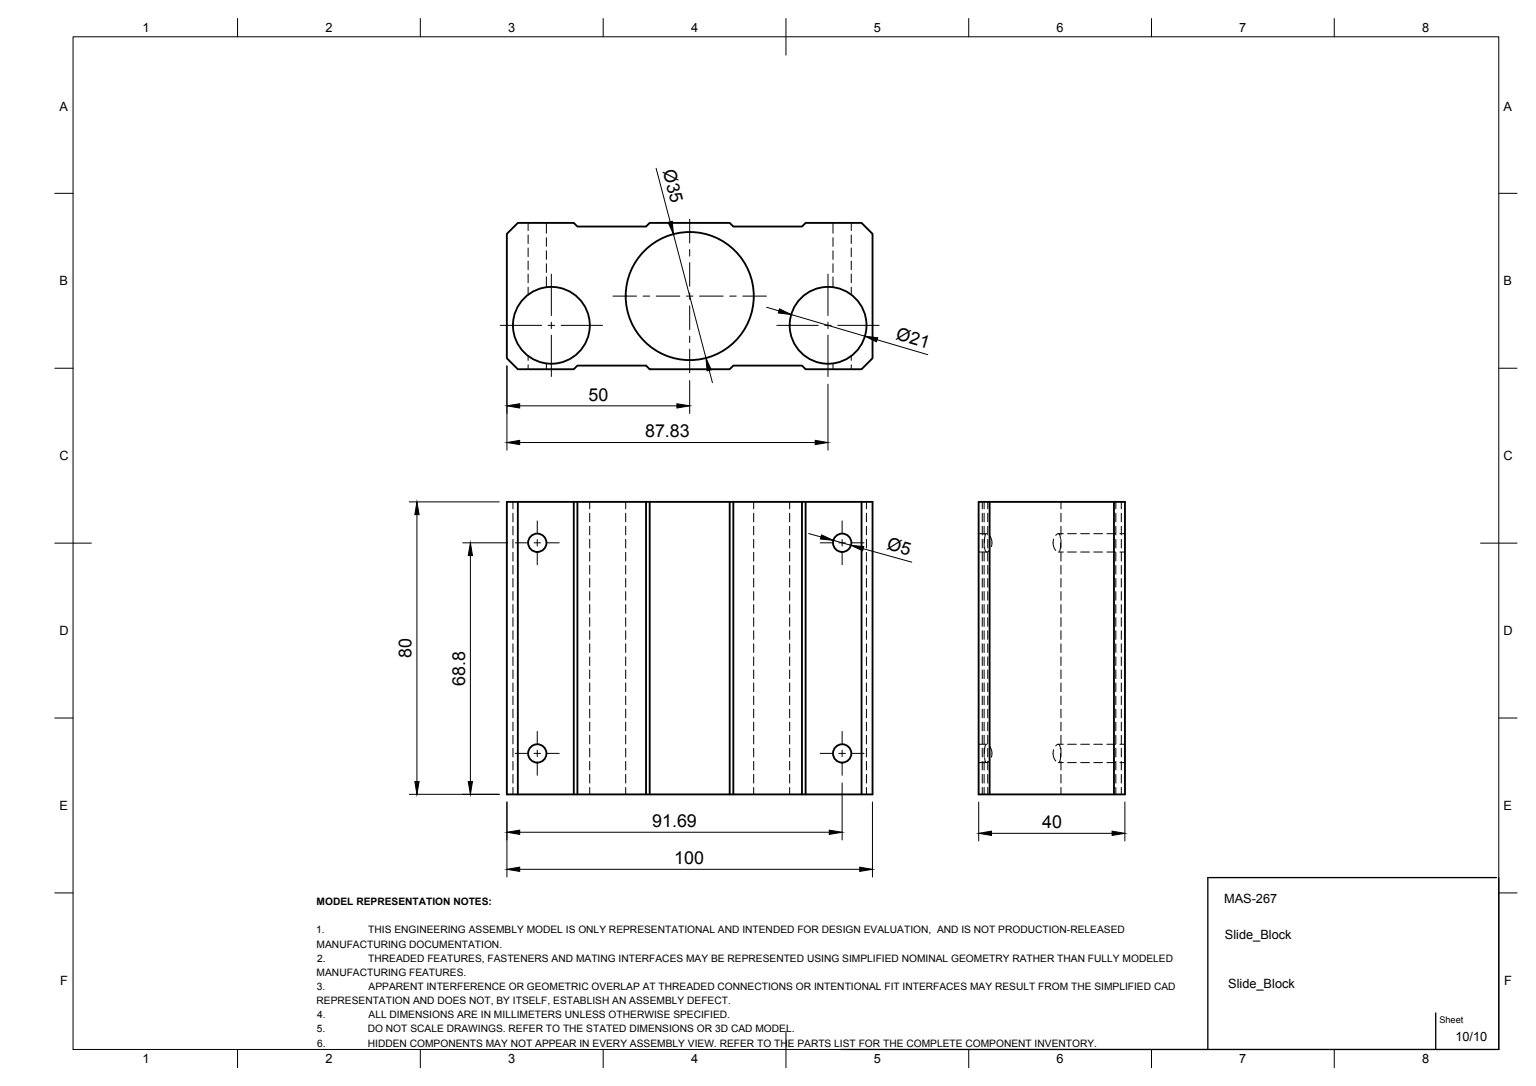
ISO-10303-21;
HEADER;
/* Generated by software containing ST-Developer
 * from STEP Tools, Inc. (www.steptools.com) 
 */

FILE_DESCRIPTION(
/* description */ (''),
/* implementation_level */ '2;1');

FILE_NAME(
/* name */ 'Slide_Block.step',
/* time_stamp */ '2026-10-12T15:29:24-07:00',
/* author */ (''),
/* organization */ (''),
/* preprocessor_version */ 'ST-DEVELOPER v20.2',
/* originating_system */ 'Autodesk Translation Framework v15.15.0.0',
/* authorisation */ '');

FILE_SCHEMA (('AUTOMOTIVE_DESIGN { 1 0 10303 214 3 1 1 }'));
ENDSEC;

DATA;
#10=MECHANICAL_DESIGN_GEOMETRIC_PRESENTATION_REPRESENTATION('',(#219),#9496);
#79=B_SPLINE_CURVE_WITH_KNOTS('',3,(#8964,#8965,#8966,#8967,#8968,#8969,
#8970,#8971,#8972,#8973),.UNSPECIFIED.,.F.,.F.,(4,2,2,2,4),(-1.57648415340294,
-1.48130138260372,-1.38611861180451,-1.27940954804234,-1.17270048428017),
 .UNSPECIFIED.);
#80=B_SPLINE_CURVE_WITH_KNOTS('',3,(#8974,#8975,#8976,#8977,#8978,#8979,
#8980,#8981,#8982,#8983,#8984,#8985,#8986,#8987,#8988,#8989,#8990,#8991,
#8992,#8993,#8994,#8995,#8996,#8997,#8998,#8999),.UNSPECIFIED.,.F.,.F.,
(4,2,2,2,2,2,2,2,2,2,2,2,4),(-1.17270048428017,-1.07435447096729,-0.976008457654416,
-0.882125267177943,-0.78824207670147,-0.694358886224997,-0.600475695748524,
-0.502129682435648,-0.403783669122773,-0.297074605360601,-0.190365541598429,
-0.0951827707992146,0.),.UNSPECIFIED.);
#81=B_SPLINE_CURVE_WITH_KNOTS('',3,(#9003,#9004,#9005,#9006,#9007,#9008,
#9009,#9010,#9011,#9012,#9013,#9014,#9015,#9016,#9017,#9018,#9019,#9020,
#9021,#9022,#9023,#9024,#9025,#9026,#9027,#9028),.UNSPECIFIED.,.F.,.F.,
(4,2,2,2,2,2,2,2,2,2,2,2,4),(-1.57648415340294,-1.48130138260372,-1.38611861180451,
-1.27940954804234,-1.17270048428017,-1.07435447096729,-0.976008457654416,
-0.882125267177943,-0.78824207670147,-0.694358886224997,-0.600475695748524,
-0.502129682435648,-0.403783669122773),.UNSPECIFIED.);
#82=B_SPLINE_CURVE_WITH_KNOTS('',3,(#9029,#9030,#9031,#9032,#9033,#9034,
#9035,#9036,#9037,#9038),.UNSPECIFIED.,.F.,.F.,(4,2,2,2,4),(-0.403783669122773,
-0.297074605360601,-0.190365541598429,-0.0951827707992147,0.),
 .UNSPECIFIED.);
#83=B_SPLINE_CURVE_WITH_KNOTS('',3,(#9048,#9049,#9050,#9051,#9052,#9053,
#9054,#9055,#9056,#9057,#9058,#9059,#9060,#9061,#9062,#9063,#9064,#9065,
#9066,#9067,#9068,#9069,#9070,#9071,#9072,#9073),.UNSPECIFIED.,.F.,.F.,
(4,2,2,2,2,2,2,2,2,2,2,2,4),(-1.57648415340294,-1.48130138260372,-1.38611861180451,
-1.27940954804234,-1.17270048428017,-1.07435447096729,-0.976008457654416,
-0.882125267177943,-0.78824207670147,-0.694358886224997,-0.600475695748524,
-0.502129682435648,-0.403783669122773),.UNSPECIFIED.);
#84=B_SPLINE_CURVE_WITH_KNOTS('',3,(#9074,#9075,#9076,#9077,#9078,#9079,
#9080,#9081,#9082,#9083),.UNSPECIFIED.,.F.,.F.,(4,2,2,2,4),(-0.403783669122773,
-0.297074605360601,-0.190365541598429,-0.0951827707992146,0.),
 .UNSPECIFIED.);
#85=B_SPLINE_CURVE_WITH_KNOTS('',3,(#9087,#9088,#9089,#9090,#9091,#9092,
#9093,#9094,#9095,#9096),.UNSPECIFIED.,.F.,.F.,(4,2,2,2,4),(-1.57648415340294,
-1.48130138260372,-1.38611861180451,-1.27940954804234,-1.17270048428017),
 .UNSPECIFIED.);
#86=B_SPLINE_CURVE_WITH_KNOTS('',3,(#9097,#9098,#9099,#9100,#9101,#9102,
#9103,#9104,#9105,#9106,#9107,#9108,#9109,#9110,#9111,#9112,#9113,#9114,
#9115,#9116,#9117,#9118,#9119,#9120,#9121,#9122),.UNSPECIFIED.,.F.,.F.,
(4,2,2,2,2,2,2,2,2,2,2,2,4),(-1.17270048428017,-1.07435447096729,-0.976008457654416,
-0.882125267177943,-0.78824207670147,-0.694358886224997,-0.600475695748524,
-0.502129682435648,-0.403783669122773,-0.297074605360601,-0.190365541598429,
-0.0951827707992147,0.),.UNSPECIFIED.);
#87=B_SPLINE_CURVE_WITH_KNOTS('',3,(#9132,#9133,#9134,#9135,#9136,#9137,
#9138,#9139,#9140,#9141),.UNSPECIFIED.,.F.,.F.,(4,2,2,2,4),(-1.57648415340294,
-1.48130138260372,-1.38611861180451,-1.27940954804234,-1.17270048428017),
 .UNSPECIFIED.);
#88=B_SPLINE_CURVE_WITH_KNOTS('',3,(#9142,#9143,#9144,#9145,#9146,#9147,
#9148,#9149,#9150,#9151,#9152,#9153,#9154,#9155,#9156,#9157,#9158,#9159,
#9160,#9161,#9162,#9163,#9164,#9165,#9166,#9167),.UNSPECIFIED.,.F.,.F.,
(4,2,2,2,2,2,2,2,2,2,2,2,4),(-1.17270048428017,-1.07435447096729,-0.976008457654416,
-0.882125267177943,-0.78824207670147,-0.694358886224997,-0.600475695748524,
-0.502129682435648,-0.403783669122773,-0.297074605360601,-0.190365541598429,
-0.0951827707992146,0.),.UNSPECIFIED.);
#89=B_SPLINE_CURVE_WITH_KNOTS('',3,(#9171,#9172,#9173,#9174,#9175,#9176,
#9177,#9178,#9179,#9180,#9181,#9182,#9183,#9184,#9185,#9186,#9187,#9188,
#9189,#9190,#9191,#9192,#9193,#9194,#9195,#9196),.UNSPECIFIED.,.F.,.F.,
(4,2,2,2,2,2,2,2,2,2,2,2,4),(-1.57648415340294,-1.48130138260372,-1.38611861180451,
-1.27940954804234,-1.17270048428017,-1.07435447096729,-0.976008457654416,
-0.882125267177943,-0.78824207670147,-0.694358886224997,-0.600475695748524,
-0.502129682435648,-0.403783669122773),.UNSPECIFIED.);
#90=B_SPLINE_CURVE_WITH_KNOTS('',3,(#9197,#9198,#9199,#9200,#9201,#9202,
#9203,#9204,#9205,#9206),.UNSPECIFIED.,.F.,.F.,(4,2,2,2,4),(-0.403783669122773,
-0.297074605360601,-0.190365541598429,-0.0951827707992147,0.),
 .UNSPECIFIED.);
#91=B_SPLINE_CURVE_WITH_KNOTS('',3,(#9216,#9217,#9218,#9219,#9220,#9221,
#9222,#9223,#9224,#9225,#9226,#9227,#9228,#9229,#9230,#9231,#9232,#9233,
#9234,#9235,#9236,#9237,#9238,#9239,#9240,#9241),.UNSPECIFIED.,.F.,.F.,
(4,2,2,2,2,2,2,2,2,2,2,2,4),(-1.57648415340294,-1.48130138260372,-1.38611861180451,
-1.27940954804234,-1.17270048428017,-1.07435447096729,-0.976008457654416,
-0.882125267177943,-0.78824207670147,-0.694358886224997,-0.600475695748524,
-0.502129682435648,-0.403783669122773),.UNSPECIFIED.);
#92=B_SPLINE_CURVE_WITH_KNOTS('',3,(#9242,#9243,#9244,#9245,#9246,#9247,
#9248,#9249,#9250,#9251),.UNSPECIFIED.,.F.,.F.,(4,2,2,2,4),(-0.403783669122773,
-0.297074605360601,-0.190365541598429,-0.0951827707992146,0.),
 .UNSPECIFIED.);
#93=B_SPLINE_CURVE_WITH_KNOTS('',3,(#9255,#9256,#9257,#9258,#9259,#9260,
#9261,#9262,#9263,#9264),.UNSPECIFIED.,.F.,.F.,(4,2,2,2,4),(-1.57648415340294,
-1.48130138260372,-1.38611861180451,-1.27940954804234,-1.17270048428017),
 .UNSPECIFIED.);
#94=B_SPLINE_CURVE_WITH_KNOTS('',3,(#9265,#9266,#9267,#9268,#9269,#9270,
#9271,#9272,#9273,#9274,#9275,#9276,#9277,#9278,#9279,#9280,#9281,#9282,
#9283,#9284,#9285,#9286,#9287,#9288,#9289,#9290),.UNSPECIFIED.,.F.,.F.,
(4,2,2,2,2,2,2,2,2,2,2,2,4),(-1.17270048428017,-1.07435447096729,-0.976008457654416,
-0.882125267177943,-0.78824207670147,-0.694358886224997,-0.600475695748524,
-0.502129682435648,-0.403783669122773,-0.297074605360601,-0.190365541598429,
-0.0951827707992147,0.),.UNSPECIFIED.);
#153=SHAPE_REPRESENTATION_RELATIONSHIP('SRR','None',#9547,#162);
#162=ADVANCED_BREP_SHAPE_REPRESENTATION('',(#276),#9495);
#219=STYLED_ITEM('',(#9593),#276);
#276=MANIFOLD_SOLID_BREP('Body1',#5021);
#460=FACE_BOUND('',#1388,.T.);
#461=FACE_BOUND('',#1389,.T.);
#462=FACE_BOUND('',#1392,.T.);
#463=FACE_BOUND('',#1393,.T.);
#464=FACE_BOUND('',#1394,.T.);
#465=FACE_BOUND('',#1399,.T.);
#466=FACE_BOUND('',#1400,.T.);
#467=FACE_BOUND('',#1401,.T.);
#468=FACE_BOUND('',#1403,.T.);
#469=FACE_BOUND('',#1404,.T.);
#470=FACE_BOUND('',#1409,.T.);
#471=FACE_BOUND('',#1410,.T.);
#472=FACE_BOUND('',#1416,.T.);
#473=FACE_BOUND('',#1417,.T.);
#474=FACE_BOUND('',#1419,.T.);
#475=FACE_BOUND('',#1420,.T.);
#476=FACE_BOUND('',#1421,.T.);
#477=FACE_BOUND('',#1422,.T.);
#478=FACE_BOUND('',#1424,.T.);
#479=FACE_BOUND('',#1425,.T.);
#480=FACE_BOUND('',#1426,.T.);
#481=FACE_BOUND('',#1427,.T.);
#596=PLANE('',#5774);
#597=PLANE('',#5775);
#598=PLANE('',#5776);
#599=PLANE('',#5777);
#600=PLANE('',#5778);
#601=PLANE('',#5779);
#602=PLANE('',#5783);
#603=PLANE('',#5784);
#604=PLANE('',#5785);
#605=PLANE('',#5786);
#606=PLANE('',#5790);
#607=PLANE('',#5791);
#608=PLANE('',#5792);
#609=PLANE('',#5793);
#610=PLANE('',#5794);
#611=PLANE('',#5795);
#612=PLANE('',#5796);
#613=PLANE('',#5797);
#614=PLANE('',#5798);
#615=PLANE('',#5799);
#616=PLANE('',#5803);
#617=PLANE('',#5804);
#618=PLANE('',#5805);
#619=PLANE('',#5806);
#620=PLANE('',#5807);
#621=PLANE('',#5808);
#917=FACE_OUTER_BOUND('',#1376,.T.);
#918=FACE_OUTER_BOUND('',#1377,.T.);
#919=FACE_OUTER_BOUND('',#1378,.T.);
#920=FACE_OUTER_BOUND('',#1379,.T.);
#921=FACE_OUTER_BOUND('',#1380,.T.);
#922=FACE_OUTER_BOUND('',#1381,.T.);
#923=FACE_OUTER_BOUND('',#1382,.T.);
#924=FACE_OUTER_BOUND('',#1383,.T.);
#925=FACE_OUTER_BOUND('',#1384,.T.);
#926=FACE_OUTER_BOUND('',#1385,.T.);
#927=FACE_OUTER_BOUND('',#1386,.T.);
#928=FACE_OUTER_BOUND('',#1387,.T.);
#929=FACE_OUTER_BOUND('',#1390,.T.);
#930=FACE_OUTER_BOUND('',#1391,.T.);
#931=FACE_OUTER_BOUND('',#1395,.T.);
#932=FACE_OUTER_BOUND('',#1396,.T.);
#933=FACE_OUTER_BOUND('',#1397,.T.);
#934=FACE_OUTER_BOUND('',#1398,.T.);
#935=FACE_OUTER_BOUND('',#1402,.T.);
#936=FACE_OUTER_BOUND('',#1405,.T.);
#937=FACE_OUTER_BOUND('',#1406,.T.);
#938=FACE_OUTER_BOUND('',#1407,.T.);
#939=FACE_OUTER_BOUND('',#1408,.T.);
#940=FACE_OUTER_BOUND('',#1411,.T.);
#941=FACE_OUTER_BOUND('',#1412,.T.);
#942=FACE_OUTER_BOUND('',#1413,.T.);
#943=FACE_OUTER_BOUND('',#1414,.T.);
#944=FACE_OUTER_BOUND('',#1415,.T.);
#945=FACE_OUTER_BOUND('',#1418,.T.);
#946=FACE_OUTER_BOUND('',#1423,.T.);
#947=FACE_OUTER_BOUND('',#1428,.T.);
#948=FACE_OUTER_BOUND('',#1429,.T.);
#949=FACE_OUTER_BOUND('',#1430,.T.);
#950=FACE_OUTER_BOUND('',#1431,.T.);
#951=FACE_OUTER_BOUND('',#1432,.T.);
#952=FACE_OUTER_BOUND('',#1433,.T.);
#953=FACE_OUTER_BOUND('',#1434,.T.);
#1376=EDGE_LOOP('',(#4319,#4320,#4321,#4322,#4323));
#1377=EDGE_LOOP('',(#4324,#4325,#4326,#4327,#4328));
#1378=EDGE_LOOP('',(#4329,#4330,#4331,#4332,#4333));
#1379=EDGE_LOOP('',(#4334,#4335,#4336,#4337,#4338));
#1380=EDGE_LOOP('',(#4339,#4340,#4341,#4342,#4343));
#1381=EDGE_LOOP('',(#4344,#4345,#4346,#4347,#4348));
#1382=EDGE_LOOP('',(#4349,#4350,#4351,#4352,#4353));
#1383=EDGE_LOOP('',(#4354,#4355,#4356,#4357,#4358));
#1384=EDGE_LOOP('',(#4359,#4360,#4361,#4362));
#1385=EDGE_LOOP('',(#4363,#4364,#4365,#4366));
#1386=EDGE_LOOP('',(#4367,#4368,#4369,#4370));
#1387=EDGE_LOOP('',(#4371,#4372,#4373,#4374));
#1388=EDGE_LOOP('',(#4375));
#1389=EDGE_LOOP('',(#4376));
#1390=EDGE_LOOP('',(#4377,#4378,#4379,#4380));
#1391=EDGE_LOOP('',(#4381,#4382,#4383,#4384,#4385,#4386,#4387,#4388,#4389,
#4390,#4391,#4392,#4393,#4394,#4395,#4396,#4397,#4398,#4399,#4400,#4401,
#4402,#4403,#4404));
#1392=EDGE_LOOP('',(#4405));
#1393=EDGE_LOOP('',(#4406));
#1394=EDGE_LOOP('',(#4407));
#1395=EDGE_LOOP('',(#4408,#4409,#4410,#4411));
#1396=EDGE_LOOP('',(#4412,#4413,#4414,#4415));
#1397=EDGE_LOOP('',(#4416,#4417,#4418,#4419));
#1398=EDGE_LOOP('',(#4420,#4421,#4422,#4423,#4424,#4425,#4426,#4427,#4428,
#4429,#4430,#4431,#4432,#4433,#4434,#4435,#4436,#4437,#4438,#4439,#4440,
#4441,#4442,#4443));
#1399=EDGE_LOOP('',(#4444));
#1400=EDGE_LOOP('',(#4445));
#1401=EDGE_LOOP('',(#4446));
#1402=EDGE_LOOP('',(#4447,#4448,#4449,#4450));
#1403=EDGE_LOOP('',(#4451));
#1404=EDGE_LOOP('',(#4452));
#1405=EDGE_LOOP('',(#4453,#4454,#4455,#4456));
#1406=EDGE_LOOP('',(#4457,#4458,#4459,#4460));
#1407=EDGE_LOOP('',(#4461,#4462,#4463,#4464));
#1408=EDGE_LOOP('',(#4465,#4466,#4467,#4468));
#1409=EDGE_LOOP('',(#4469));
#1410=EDGE_LOOP('',(#4470));
#1411=EDGE_LOOP('',(#4471,#4472,#4473,#4474));
#1412=EDGE_LOOP('',(#4475,#4476,#4477,#4478));
#1413=EDGE_LOOP('',(#4479,#4480,#4481,#4482));
#1414=EDGE_LOOP('',(#4483,#4484,#4485,#4486));
#1415=EDGE_LOOP('',(#4487,#4488,#4489,#4490));
#1416=EDGE_LOOP('',(#4491));
#1417=EDGE_LOOP('',(#4492));
#1418=EDGE_LOOP('',(#4493,#4494,#4495,#4496));
#1419=EDGE_LOOP('',(#4497,#4498));
#1420=EDGE_LOOP('',(#4499,#4500));
#1421=EDGE_LOOP('',(#4501,#4502));
#1422=EDGE_LOOP('',(#4503,#4504));
#1423=EDGE_LOOP('',(#4505,#4506,#4507,#4508));
#1424=EDGE_LOOP('',(#4509,#4510));
#1425=EDGE_LOOP('',(#4511,#4512));
#1426=EDGE_LOOP('',(#4513,#4514));
#1427=EDGE_LOOP('',(#4515,#4516));
#1428=EDGE_LOOP('',(#4517,#4518,#4519,#4520));
#1429=EDGE_LOOP('',(#4521,#4522,#4523,#4524));
#1430=EDGE_LOOP('',(#4525,#4526,#4527,#4528));
#1431=EDGE_LOOP('',(#4529,#4530,#4531,#4532));
#1432=EDGE_LOOP('',(#4533,#4534,#4535,#4536));
#1433=EDGE_LOOP('',(#4537,#4538,#4539,#4540));
#1434=EDGE_LOOP('',(#4541,#4542,#4543,#4544));
#1589=LINE('',#8962,#1826);
#1590=LINE('',#9040,#1827);
#1591=LINE('',#9046,#1828);
#1592=LINE('',#9124,#1829);
#1593=LINE('',#9130,#1830);
#1594=LINE('',#9208,#1831);
#1595=LINE('',#9214,#1832);
#1596=LINE('',#9292,#1833);
#1597=LINE('',#9297,#1834);
#1598=LINE('',#9299,#1835);
#1599=LINE('',#9301,#1836);
#1600=LINE('',#9302,#1837);
#1601=LINE('',#9305,#1838);
#1602=LINE('',#9307,#1839);
#1603=LINE('',#9308,#1840);
#1604=LINE('',#9311,#1841);
#1605=LINE('',#9313,#1842);
#1606=LINE('',#9314,#1843);
#1607=LINE('',#9317,#1844);
#1608=LINE('',#9319,#1845);
#1609=LINE('',#9320,#1846);
#1610=LINE('',#9323,#1847);
#1611=LINE('',#9325,#1848);
#1612=LINE('',#9326,#1849);
#1613=LINE('',#9329,#1850);
#1614=LINE('',#9331,#1851);
#1615=LINE('',#9333,#1852);
#1616=LINE('',#9335,#1853);
#1617=LINE('',#9337,#1854);
#1618=LINE('',#9339,#1855);
#1619=LINE('',#9341,#1856);
#1620=LINE('',#9343,#1857);
#1621=LINE('',#9345,#1858);
#1622=LINE('',#9347,#1859);
#1623=LINE('',#9349,#1860);
#1624=LINE('',#9351,#1861);
#1625=LINE('',#9353,#1862);
#1626=LINE('',#9355,#1863);
#1627=LINE('',#9357,#1864);
#1628=LINE('',#9359,#1865);
#1629=LINE('',#9361,#1866);
#1630=LINE('',#9363,#1867);
#1631=LINE('',#9364,#1868);
#1632=LINE('',#9373,#1869);
#1633=LINE('',#9375,#1870);
#1634=LINE('',#9376,#1871);
#1635=LINE('',#9379,#1872);
#1636=LINE('',#9380,#1873);
#1637=LINE('',#9382,#1874);
#1638=LINE('',#9385,#1875);
#1639=LINE('',#9387,#1876);
#1640=LINE('',#9389,#1877);
#1641=LINE('',#9391,#1878);
#1642=LINE('',#9393,#1879);
#1643=LINE('',#9395,#1880);
#1644=LINE('',#9397,#1881);
#1645=LINE('',#9399,#1882);
#1646=LINE('',#9401,#1883);
#1647=LINE('',#9403,#1884);
#1648=LINE('',#9405,#1885);
#1649=LINE('',#9407,#1886);
#1650=LINE('',#9409,#1887);
#1651=LINE('',#9411,#1888);
#1652=LINE('',#9413,#1889);
#1653=LINE('',#9414,#1890);
#1654=LINE('',#9422,#1891);
#1655=LINE('',#9424,#1892);
#1656=LINE('',#9425,#1893);
#1657=LINE('',#9427,#1894);
#1658=LINE('',#9429,#1895);
#1659=LINE('',#9431,#1896);
#1660=LINE('',#9433,#1897);
#1661=LINE('',#9435,#1898);
#1662=LINE('',#9436,#1899);
#1663=LINE('',#9438,#1900);
#1664=LINE('',#9441,#1901);
#1665=LINE('',#9443,#1902);
#1666=LINE('',#9445,#1903);
#1667=LINE('',#9447,#1904);
#1668=LINE('',#9449,#1905);
#1669=LINE('',#9451,#1906);
#1670=LINE('',#9454,#1907);
#1671=LINE('',#9456,#1908);
#1826=VECTOR('',#7256,2.5);
#1827=VECTOR('',#7259,2.5);
#1828=VECTOR('',#7266,2.5);
#1829=VECTOR('',#7269,2.5);
#1830=VECTOR('',#7276,2.5);
#1831=VECTOR('',#7279,2.5);
#1832=VECTOR('',#7286,2.5);
#1833=VECTOR('',#7289,2.5);
#1834=VECTOR('',#7294,10.);
#1835=VECTOR('',#7295,10.);
#1836=VECTOR('',#7296,10.);
#1837=VECTOR('',#7297,10.);
#1838=VECTOR('',#7300,10.);
#1839=VECTOR('',#7301,10.);
#1840=VECTOR('',#7302,10.);
#1841=VECTOR('',#7305,10.);
#1842=VECTOR('',#7306,10.);
#1843=VECTOR('',#7307,10.);
#1844=VECTOR('',#7310,10.);
#1845=VECTOR('',#7311,10.);
#1846=VECTOR('',#7312,10.);
#1847=VECTOR('',#7315,10.);
#1848=VECTOR('',#7316,10.);
#1849=VECTOR('',#7317,10.);
#1850=VECTOR('',#7320,10.);
#1851=VECTOR('',#7321,10.);
#1852=VECTOR('',#7322,10.);
#1853=VECTOR('',#7323,10.);
#1854=VECTOR('',#7324,10.);
#1855=VECTOR('',#7325,10.);
#1856=VECTOR('',#7326,10.);
#1857=VECTOR('',#7327,10.);
#1858=VECTOR('',#7328,10.);
#1859=VECTOR('',#7329,10.);
#1860=VECTOR('',#7330,10.);
#1861=VECTOR('',#7331,10.);
#1862=VECTOR('',#7332,10.);
#1863=VECTOR('',#7333,10.);
#1864=VECTOR('',#7334,10.);
#1865=VECTOR('',#7335,10.);
#1866=VECTOR('',#7336,10.);
#1867=VECTOR('',#7337,10.);
#1868=VECTOR('',#7338,10.);
#1869=VECTOR('',#7347,10.);
#1870=VECTOR('',#7348,10.);
#1871=VECTOR('',#7349,10.);
#1872=VECTOR('',#7352,10.);
#1873=VECTOR('',#7353,10.);
#1874=VECTOR('',#7356,10.);
#1875=VECTOR('',#7359,10.);
#1876=VECTOR('',#7360,10.);
#1877=VECTOR('',#7361,10.);
#1878=VECTOR('',#7362,10.);
#1879=VECTOR('',#7363,10.);
#1880=VECTOR('',#7364,10.);
#1881=VECTOR('',#7365,10.);
#1882=VECTOR('',#7366,10.);
#1883=VECTOR('',#7367,10.);
#1884=VECTOR('',#7368,10.);
#1885=VECTOR('',#7369,10.);
#1886=VECTOR('',#7370,10.);
#1887=VECTOR('',#7371,10.);
#1888=VECTOR('',#7372,10.);
#1889=VECTOR('',#7373,10.);
#1890=VECTOR('',#7374,10.);
#1891=VECTOR('',#7383,10.);
#1892=VECTOR('',#7386,10.);
#1893=VECTOR('',#7387,10.);
#1894=VECTOR('',#7390,10.);
#1895=VECTOR('',#7393,10.);
#1896=VECTOR('',#7396,10.);
#1897=VECTOR('',#7399,10.);
#1898=VECTOR('',#7402,10.);
#1899=VECTOR('',#7403,10.);
#1900=VECTOR('',#7406,10.);
#1901=VECTOR('',#7411,10.);
#1902=VECTOR('',#7414,10.5);
#1903=VECTOR('',#7417,10.5);
#1904=VECTOR('',#7420,17.5);
#1905=VECTOR('',#7423,10.);
#1906=VECTOR('',#7426,10.);
#1907=VECTOR('',#7431,10.);
#1908=VECTOR('',#7434,10.);
#2250=CIRCLE('',#5759,2.5);
#2251=CIRCLE('',#5761,2.5);
#2252=CIRCLE('',#5763,2.5);
#2253=CIRCLE('',#5765,2.5);
#2254=CIRCLE('',#5767,2.5);
#2255=CIRCLE('',#5769,2.5);
#2256=CIRCLE('',#5771,2.5);
#2257=CIRCLE('',#5773,2.5);
#2258=CIRCLE('',#5780,10.5);
#2259=CIRCLE('',#5781,10.5);
#2260=CIRCLE('',#5782,17.5);
#2261=CIRCLE('',#5787,10.5);
#2262=CIRCLE('',#5788,10.5);
#2263=CIRCLE('',#5789,17.5);
#2637=VERTEX_POINT('',#8959);
#2638=VERTEX_POINT('',#8961);
#2639=VERTEX_POINT('',#8963);
#2640=VERTEX_POINT('',#9001);
#2641=VERTEX_POINT('',#9002);
#2642=VERTEX_POINT('',#9039);
#2643=VERTEX_POINT('',#9043);
#2644=VERTEX_POINT('',#9045);
#2645=VERTEX_POINT('',#9047);
#2646=VERTEX_POINT('',#9085);
#2647=VERTEX_POINT('',#9086);
#2648=VERTEX_POINT('',#9123);
#2649=VERTEX_POINT('',#9127);
#2650=VERTEX_POINT('',#9129);
#2651=VERTEX_POINT('',#9131);
#2652=VERTEX_POINT('',#9169);
#2653=VERTEX_POINT('',#9170);
#2654=VERTEX_POINT('',#9207);
#2655=VERTEX_POINT('',#9211);
#2656=VERTEX_POINT('',#9213);
#2657=VERTEX_POINT('',#9215);
#2658=VERTEX_POINT('',#9253);
#2659=VERTEX_POINT('',#9254);
#2660=VERTEX_POINT('',#9291);
#2661=VERTEX_POINT('',#9295);
#2662=VERTEX_POINT('',#9296);
#2663=VERTEX_POINT('',#9298);
#2664=VERTEX_POINT('',#9300);
#2665=VERTEX_POINT('',#9304);
#2666=VERTEX_POINT('',#9306);
#2667=VERTEX_POINT('',#9310);
#2668=VERTEX_POINT('',#9312);
#2669=VERTEX_POINT('',#9316);
#2670=VERTEX_POINT('',#9318);
#2671=VERTEX_POINT('',#9322);
#2672=VERTEX_POINT('',#9324);
#2673=VERTEX_POINT('',#9328);
#2674=VERTEX_POINT('',#9330);
#2675=VERTEX_POINT('',#9332);
#2676=VERTEX_POINT('',#9334);
#2677=VERTEX_POINT('',#9336);
#2678=VERTEX_POINT('',#9338);
#2679=VERTEX_POINT('',#9340);
#2680=VERTEX_POINT('',#9342);
#2681=VERTEX_POINT('',#9344);
#2682=VERTEX_POINT('',#9346);
#2683=VERTEX_POINT('',#9348);
#2684=VERTEX_POINT('',#9350);
#2685=VERTEX_POINT('',#9352);
#2686=VERTEX_POINT('',#9354);
#2687=VERTEX_POINT('',#9356);
#2688=VERTEX_POINT('',#9358);
#2689=VERTEX_POINT('',#9360);
#2690=VERTEX_POINT('',#9362);
#2691=VERTEX_POINT('',#9365);
#2692=VERTEX_POINT('',#9367);
#2693=VERTEX_POINT('',#9369);
#2694=VERTEX_POINT('',#9372);
#2695=VERTEX_POINT('',#9374);
#2696=VERTEX_POINT('',#9378);
#2697=VERTEX_POINT('',#9384);
#2698=VERTEX_POINT('',#9386);
#2699=VERTEX_POINT('',#9388);
#2700=VERTEX_POINT('',#9390);
#2701=VERTEX_POINT('',#9392);
#2702=VERTEX_POINT('',#9394);
#2703=VERTEX_POINT('',#9396);
#2704=VERTEX_POINT('',#9398);
#2705=VERTEX_POINT('',#9400);
#2706=VERTEX_POINT('',#9402);
#2707=VERTEX_POINT('',#9404);
#2708=VERTEX_POINT('',#9406);
#2709=VERTEX_POINT('',#9408);
#2710=VERTEX_POINT('',#9410);
#2711=VERTEX_POINT('',#9412);
#2712=VERTEX_POINT('',#9415);
#2713=VERTEX_POINT('',#9417);
#2714=VERTEX_POINT('',#9419);
#3212=EDGE_CURVE('',#2637,#2637,#2250,.T.);
#3213=EDGE_CURVE('',#2637,#2638,#1589,.T.);
#3214=EDGE_CURVE('',#2639,#2638,#79,.T.);
#3215=EDGE_CURVE('',#2638,#2639,#80,.T.);
#3216=EDGE_CURVE('',#2640,#2641,#81,.T.);
#3217=EDGE_CURVE('',#2641,#2640,#82,.T.);
#3218=EDGE_CURVE('',#2641,#2642,#1590,.T.);
#3219=EDGE_CURVE('',#2642,#2642,#2251,.T.);
#3220=EDGE_CURVE('',#2643,#2643,#2252,.T.);
#3221=EDGE_CURVE('',#2643,#2644,#1591,.T.);
#3222=EDGE_CURVE('',#2645,#2644,#83,.T.);
#3223=EDGE_CURVE('',#2644,#2645,#84,.T.);
#3224=EDGE_CURVE('',#2646,#2647,#85,.T.);
#3225=EDGE_CURVE('',#2647,#2646,#86,.T.);
#3226=EDGE_CURVE('',#2647,#2648,#1592,.T.);
#3227=EDGE_CURVE('',#2648,#2648,#2253,.T.);
#3228=EDGE_CURVE('',#2649,#2649,#2254,.T.);
#3229=EDGE_CURVE('',#2649,#2650,#1593,.T.);
#3230=EDGE_CURVE('',#2651,#2650,#87,.T.);
#3231=EDGE_CURVE('',#2650,#2651,#88,.T.);
#3232=EDGE_CURVE('',#2652,#2653,#89,.T.);
#3233=EDGE_CURVE('',#2653,#2652,#90,.T.);
#3234=EDGE_CURVE('',#2653,#2654,#1594,.T.);
#3235=EDGE_CURVE('',#2654,#2654,#2255,.T.);
#3236=EDGE_CURVE('',#2655,#2655,#2256,.T.);
#3237=EDGE_CURVE('',#2655,#2656,#1595,.T.);
#3238=EDGE_CURVE('',#2657,#2656,#91,.T.);
#3239=EDGE_CURVE('',#2656,#2657,#92,.T.);
#3240=EDGE_CURVE('',#2658,#2659,#93,.T.);
#3241=EDGE_CURVE('',#2659,#2658,#94,.T.);
#3242=EDGE_CURVE('',#2659,#2660,#1596,.T.);
#3243=EDGE_CURVE('',#2660,#2660,#2257,.T.);
#3244=EDGE_CURVE('',#2661,#2662,#1597,.T.);
#3245=EDGE_CURVE('',#2661,#2663,#1598,.T.);
#3246=EDGE_CURVE('',#2664,#2663,#1599,.T.);
#3247=EDGE_CURVE('',#2662,#2664,#1600,.T.);
#3248=EDGE_CURVE('',#2665,#2661,#1601,.T.);
#3249=EDGE_CURVE('',#2665,#2666,#1602,.T.);
#3250=EDGE_CURVE('',#2663,#2666,#1603,.T.);
#3251=EDGE_CURVE('',#2667,#2665,#1604,.T.);
#3252=EDGE_CURVE('',#2668,#2667,#1605,.T.);
#3253=EDGE_CURVE('',#2666,#2668,#1606,.T.);
#3254=EDGE_CURVE('',#2664,#2669,#1607,.T.);
#3255=EDGE_CURVE('',#2670,#2669,#1608,.T.);
#3256=EDGE_CURVE('',#2670,#2662,#1609,.T.);
#3257=EDGE_CURVE('',#2667,#2671,#1610,.T.);
#3258=EDGE_CURVE('',#2671,#2672,#1611,.T.);
#3259=EDGE_CURVE('',#2672,#2668,#1612,.T.);
#3260=EDGE_CURVE('',#2673,#2670,#1613,.T.);
#3261=EDGE_CURVE('',#2673,#2674,#1614,.T.);
#3262=EDGE_CURVE('',#2675,#2674,#1615,.T.);
#3263=EDGE_CURVE('',#2676,#2675,#1616,.T.);
#3264=EDGE_CURVE('',#2676,#2677,#1617,.T.);
#3265=EDGE_CURVE('',#2677,#2678,#1618,.T.);
#3266=EDGE_CURVE('',#2678,#2679,#1619,.T.);
#3267=EDGE_CURVE('',#2680,#2679,#1620,.T.);
#3268=EDGE_CURVE('',#2680,#2681,#1621,.T.);
#3269=EDGE_CURVE('',#2681,#2682,#1622,.T.);
#3270=EDGE_CURVE('',#2682,#2683,#1623,.T.);
#3271=EDGE_CURVE('',#2684,#2683,#1624,.T.);
#3272=EDGE_CURVE('',#2685,#2684,#1625,.T.);
#3273=EDGE_CURVE('',#2686,#2685,#1626,.T.);
#3274=EDGE_CURVE('',#2687,#2686,#1627,.T.);
#3275=EDGE_CURVE('',#2688,#2687,#1628,.T.);
#3276=EDGE_CURVE('',#2688,#2689,#1629,.T.);
#3277=EDGE_CURVE('',#2689,#2690,#1630,.T.);
#3278=EDGE_CURVE('',#2690,#2671,#1631,.T.);
#3279=EDGE_CURVE('',#2691,#2691,#2258,.T.);
#3280=EDGE_CURVE('',#2692,#2692,#2259,.T.);
#3281=EDGE_CURVE('',#2693,#2693,#2260,.T.);
#3282=EDGE_CURVE('',#2694,#2688,#1632,.T.);
#3283=EDGE_CURVE('',#2695,#2694,#1633,.T.);
#3284=EDGE_CURVE('',#2689,#2695,#1634,.T.);
#3285=EDGE_CURVE('',#2696,#2695,#1635,.T.);
#3286=EDGE_CURVE('',#2690,#2696,#1636,.T.);
#3287=EDGE_CURVE('',#2672,#2696,#1637,.T.);
#3288=EDGE_CURVE('',#2697,#2694,#1638,.T.);
#3289=EDGE_CURVE('',#2698,#2697,#1639,.T.);
#3290=EDGE_CURVE('',#2699,#2698,#1640,.T.);
#3291=EDGE_CURVE('',#2700,#2699,#1641,.T.);
#3292=EDGE_CURVE('',#2701,#2700,#1642,.T.);
#3293=EDGE_CURVE('',#2701,#2702,#1643,.T.);
#3294=EDGE_CURVE('',#2702,#2703,#1644,.T.);
#3295=EDGE_CURVE('',#2703,#2704,#1645,.T.);
#3296=EDGE_CURVE('',#2705,#2704,#1646,.T.);
#3297=EDGE_CURVE('',#2705,#2706,#1647,.T.);
#3298=EDGE_CURVE('',#2706,#2707,#1648,.T.);
#3299=EDGE_CURVE('',#2707,#2708,#1649,.T.);
#3300=EDGE_CURVE('',#2709,#2708,#1650,.T.);
#3301=EDGE_CURVE('',#2710,#2709,#1651,.T.);
#3302=EDGE_CURVE('',#2711,#2710,#1652,.T.);
#3303=EDGE_CURVE('',#2669,#2711,#1653,.T.);
#3304=EDGE_CURVE('',#2712,#2712,#2261,.T.);
#3305=EDGE_CURVE('',#2713,#2713,#2262,.T.);
#3306=EDGE_CURVE('',#2714,#2714,#2263,.T.);
#3307=EDGE_CURVE('',#2697,#2687,#1654,.T.);
#3308=EDGE_CURVE('',#2708,#2676,#1655,.T.);
#3309=EDGE_CURVE('',#2677,#2707,#1656,.T.);
#3310=EDGE_CURVE('',#2678,#2706,#1657,.T.);
#3311=EDGE_CURVE('',#2679,#2705,#1658,.T.);
#3312=EDGE_CURVE('',#2709,#2675,#1659,.T.);
#3313=EDGE_CURVE('',#2704,#2680,#1660,.T.);
#3314=EDGE_CURVE('',#2682,#2702,#1661,.T.);
#3315=EDGE_CURVE('',#2683,#2701,#1662,.T.);
#3316=EDGE_CURVE('',#2681,#2703,#1663,.T.);
#3317=EDGE_CURVE('',#2684,#2700,#1664,.T.);
#3318=EDGE_CURVE('',#2691,#2712,#1665,.T.);
#3319=EDGE_CURVE('',#2713,#2692,#1666,.T.);
#3320=EDGE_CURVE('',#2714,#2693,#1667,.T.);
#3321=EDGE_CURVE('',#2686,#2698,#1668,.T.);
#3322=EDGE_CURVE('',#2699,#2685,#1669,.T.);
#3323=EDGE_CURVE('',#2711,#2673,#1670,.T.);
#3324=EDGE_CURVE('',#2674,#2710,#1671,.T.);
#4319=ORIENTED_EDGE('',*,*,#3212,.F.);
#4320=ORIENTED_EDGE('',*,*,#3213,.T.);
#4321=ORIENTED_EDGE('',*,*,#3214,.F.);
#4322=ORIENTED_EDGE('',*,*,#3215,.F.);
#4323=ORIENTED_EDGE('',*,*,#3213,.F.);
#4324=ORIENTED_EDGE('',*,*,#3216,.F.);
#4325=ORIENTED_EDGE('',*,*,#3217,.F.);
#4326=ORIENTED_EDGE('',*,*,#3218,.T.);
#4327=ORIENTED_EDGE('',*,*,#3219,.F.);
#4328=ORIENTED_EDGE('',*,*,#3218,.F.);
#4329=ORIENTED_EDGE('',*,*,#3220,.F.);
#4330=ORIENTED_EDGE('',*,*,#3221,.T.);
#4331=ORIENTED_EDGE('',*,*,#3222,.F.);
#4332=ORIENTED_EDGE('',*,*,#3223,.F.);
#4333=ORIENTED_EDGE('',*,*,#3221,.F.);
#4334=ORIENTED_EDGE('',*,*,#3224,.F.);
#4335=ORIENTED_EDGE('',*,*,#3225,.F.);
#4336=ORIENTED_EDGE('',*,*,#3226,.T.);
#4337=ORIENTED_EDGE('',*,*,#3227,.F.);
#4338=ORIENTED_EDGE('',*,*,#3226,.F.);
#4339=ORIENTED_EDGE('',*,*,#3228,.F.);
#4340=ORIENTED_EDGE('',*,*,#3229,.T.);
#4341=ORIENTED_EDGE('',*,*,#3230,.F.);
#4342=ORIENTED_EDGE('',*,*,#3231,.F.);
#4343=ORIENTED_EDGE('',*,*,#3229,.F.);
#4344=ORIENTED_EDGE('',*,*,#3232,.F.);
#4345=ORIENTED_EDGE('',*,*,#3233,.F.);
#4346=ORIENTED_EDGE('',*,*,#3234,.T.);
#4347=ORIENTED_EDGE('',*,*,#3235,.F.);
#4348=ORIENTED_EDGE('',*,*,#3234,.F.);
#4349=ORIENTED_EDGE('',*,*,#3236,.F.);
#4350=ORIENTED_EDGE('',*,*,#3237,.T.);
#4351=ORIENTED_EDGE('',*,*,#3238,.F.);
#4352=ORIENTED_EDGE('',*,*,#3239,.F.);
#4353=ORIENTED_EDGE('',*,*,#3237,.F.);
#4354=ORIENTED_EDGE('',*,*,#3240,.F.);
#4355=ORIENTED_EDGE('',*,*,#3241,.F.);
#4356=ORIENTED_EDGE('',*,*,#3242,.T.);
#4357=ORIENTED_EDGE('',*,*,#3243,.F.);
#4358=ORIENTED_EDGE('',*,*,#3242,.F.);
#4359=ORIENTED_EDGE('',*,*,#3244,.F.);
#4360=ORIENTED_EDGE('',*,*,#3245,.T.);
#4361=ORIENTED_EDGE('',*,*,#3246,.F.);
#4362=ORIENTED_EDGE('',*,*,#3247,.F.);
#4363=ORIENTED_EDGE('',*,*,#3248,.F.);
#4364=ORIENTED_EDGE('',*,*,#3249,.T.);
#4365=ORIENTED_EDGE('',*,*,#3250,.F.);
#4366=ORIENTED_EDGE('',*,*,#3245,.F.);
#4367=ORIENTED_EDGE('',*,*,#3251,.F.);
#4368=ORIENTED_EDGE('',*,*,#3252,.F.);
#4369=ORIENTED_EDGE('',*,*,#3253,.F.);
#4370=ORIENTED_EDGE('',*,*,#3249,.F.);
#4371=ORIENTED_EDGE('',*,*,#3247,.T.);
#4372=ORIENTED_EDGE('',*,*,#3254,.T.);
#4373=ORIENTED_EDGE('',*,*,#3255,.F.);
#4374=ORIENTED_EDGE('',*,*,#3256,.T.);
#4375=ORIENTED_EDGE('',*,*,#3219,.T.);
#4376=ORIENTED_EDGE('',*,*,#3235,.T.);
#4377=ORIENTED_EDGE('',*,*,#3252,.T.);
#4378=ORIENTED_EDGE('',*,*,#3257,.T.);
#4379=ORIENTED_EDGE('',*,*,#3258,.T.);
#4380=ORIENTED_EDGE('',*,*,#3259,.T.);
#4381=ORIENTED_EDGE('',*,*,#3251,.T.);
#4382=ORIENTED_EDGE('',*,*,#3248,.T.);
#4383=ORIENTED_EDGE('',*,*,#3244,.T.);
#4384=ORIENTED_EDGE('',*,*,#3256,.F.);
#4385=ORIENTED_EDGE('',*,*,#3260,.F.);
#4386=ORIENTED_EDGE('',*,*,#3261,.T.);
#4387=ORIENTED_EDGE('',*,*,#3262,.F.);
#4388=ORIENTED_EDGE('',*,*,#3263,.F.);
#4389=ORIENTED_EDGE('',*,*,#3264,.T.);
#4390=ORIENTED_EDGE('',*,*,#3265,.T.);
#4391=ORIENTED_EDGE('',*,*,#3266,.T.);
#4392=ORIENTED_EDGE('',*,*,#3267,.F.);
#4393=ORIENTED_EDGE('',*,*,#3268,.T.);
#4394=ORIENTED_EDGE('',*,*,#3269,.T.);
#4395=ORIENTED_EDGE('',*,*,#3270,.T.);
#4396=ORIENTED_EDGE('',*,*,#3271,.F.);
#4397=ORIENTED_EDGE('',*,*,#3272,.F.);
#4398=ORIENTED_EDGE('',*,*,#3273,.F.);
#4399=ORIENTED_EDGE('',*,*,#3274,.F.);
#4400=ORIENTED_EDGE('',*,*,#3275,.F.);
#4401=ORIENTED_EDGE('',*,*,#3276,.T.);
#4402=ORIENTED_EDGE('',*,*,#3277,.T.);
#4403=ORIENTED_EDGE('',*,*,#3278,.T.);
#4404=ORIENTED_EDGE('',*,*,#3257,.F.);
#4405=ORIENTED_EDGE('',*,*,#3279,.T.);
#4406=ORIENTED_EDGE('',*,*,#3280,.T.);
#4407=ORIENTED_EDGE('',*,*,#3281,.T.);
#4408=ORIENTED_EDGE('',*,*,#3276,.F.);
#4409=ORIENTED_EDGE('',*,*,#3282,.F.);
#4410=ORIENTED_EDGE('',*,*,#3283,.F.);
#4411=ORIENTED_EDGE('',*,*,#3284,.F.);
#4412=ORIENTED_EDGE('',*,*,#3277,.F.);
#4413=ORIENTED_EDGE('',*,*,#3284,.T.);
#4414=ORIENTED_EDGE('',*,*,#3285,.F.);
#4415=ORIENTED_EDGE('',*,*,#3286,.F.);
#4416=ORIENTED_EDGE('',*,*,#3278,.F.);
#4417=ORIENTED_EDGE('',*,*,#3286,.T.);
#4418=ORIENTED_EDGE('',*,*,#3287,.F.);
#4419=ORIENTED_EDGE('',*,*,#3258,.F.);
#4420=ORIENTED_EDGE('',*,*,#3253,.T.);
#4421=ORIENTED_EDGE('',*,*,#3259,.F.);
#4422=ORIENTED_EDGE('',*,*,#3287,.T.);
#4423=ORIENTED_EDGE('',*,*,#3285,.T.);
#4424=ORIENTED_EDGE('',*,*,#3283,.T.);
#4425=ORIENTED_EDGE('',*,*,#3288,.F.);
#4426=ORIENTED_EDGE('',*,*,#3289,.F.);
#4427=ORIENTED_EDGE('',*,*,#3290,.F.);
#4428=ORIENTED_EDGE('',*,*,#3291,.F.);
#4429=ORIENTED_EDGE('',*,*,#3292,.F.);
#4430=ORIENTED_EDGE('',*,*,#3293,.T.);
#4431=ORIENTED_EDGE('',*,*,#3294,.T.);
#4432=ORIENTED_EDGE('',*,*,#3295,.T.);
#4433=ORIENTED_EDGE('',*,*,#3296,.F.);
#4434=ORIENTED_EDGE('',*,*,#3297,.T.);
#4435=ORIENTED_EDGE('',*,*,#3298,.T.);
#4436=ORIENTED_EDGE('',*,*,#3299,.T.);
#4437=ORIENTED_EDGE('',*,*,#3300,.F.);
#4438=ORIENTED_EDGE('',*,*,#3301,.F.);
#4439=ORIENTED_EDGE('',*,*,#3302,.F.);
#4440=ORIENTED_EDGE('',*,*,#3303,.F.);
#4441=ORIENTED_EDGE('',*,*,#3254,.F.);
#4442=ORIENTED_EDGE('',*,*,#3246,.T.);
#4443=ORIENTED_EDGE('',*,*,#3250,.T.);
#4444=ORIENTED_EDGE('',*,*,#3304,.T.);
#4445=ORIENTED_EDGE('',*,*,#3305,.T.);
#4446=ORIENTED_EDGE('',*,*,#3306,.T.);
#4447=ORIENTED_EDGE('',*,*,#3282,.T.);
#4448=ORIENTED_EDGE('',*,*,#3275,.T.);
#4449=ORIENTED_EDGE('',*,*,#3307,.F.);
#4450=ORIENTED_EDGE('',*,*,#3288,.T.);
#4451=ORIENTED_EDGE('',*,*,#3227,.T.);
#4452=ORIENTED_EDGE('',*,*,#3243,.T.);
#4453=ORIENTED_EDGE('',*,*,#3264,.F.);
#4454=ORIENTED_EDGE('',*,*,#3308,.F.);
#4455=ORIENTED_EDGE('',*,*,#3299,.F.);
#4456=ORIENTED_EDGE('',*,*,#3309,.F.);
#4457=ORIENTED_EDGE('',*,*,#3265,.F.);
#4458=ORIENTED_EDGE('',*,*,#3309,.T.);
#4459=ORIENTED_EDGE('',*,*,#3298,.F.);
#4460=ORIENTED_EDGE('',*,*,#3310,.F.);
#4461=ORIENTED_EDGE('',*,*,#3266,.F.);
#4462=ORIENTED_EDGE('',*,*,#3310,.T.);
#4463=ORIENTED_EDGE('',*,*,#3297,.F.);
#4464=ORIENTED_EDGE('',*,*,#3311,.F.);
#4465=ORIENTED_EDGE('',*,*,#3308,.T.);
#4466=ORIENTED_EDGE('',*,*,#3263,.T.);
#4467=ORIENTED_EDGE('',*,*,#3312,.F.);
#4468=ORIENTED_EDGE('',*,*,#3300,.T.);
#4469=ORIENTED_EDGE('',*,*,#3212,.T.);
#4470=ORIENTED_EDGE('',*,*,#3228,.T.);
#4471=ORIENTED_EDGE('',*,*,#3311,.T.);
#4472=ORIENTED_EDGE('',*,*,#3296,.T.);
#4473=ORIENTED_EDGE('',*,*,#3313,.T.);
#4474=ORIENTED_EDGE('',*,*,#3267,.T.);
#4475=ORIENTED_EDGE('',*,*,#3270,.F.);
#4476=ORIENTED_EDGE('',*,*,#3314,.T.);
#4477=ORIENTED_EDGE('',*,*,#3293,.F.);
#4478=ORIENTED_EDGE('',*,*,#3315,.F.);
#4479=ORIENTED_EDGE('',*,*,#3269,.F.);
#4480=ORIENTED_EDGE('',*,*,#3316,.T.);
#4481=ORIENTED_EDGE('',*,*,#3294,.F.);
#4482=ORIENTED_EDGE('',*,*,#3314,.F.);
#4483=ORIENTED_EDGE('',*,*,#3268,.F.);
#4484=ORIENTED_EDGE('',*,*,#3313,.F.);
#4485=ORIENTED_EDGE('',*,*,#3295,.F.);
#4486=ORIENTED_EDGE('',*,*,#3316,.F.);
#4487=ORIENTED_EDGE('',*,*,#3315,.T.);
#4488=ORIENTED_EDGE('',*,*,#3292,.T.);
#4489=ORIENTED_EDGE('',*,*,#3317,.F.);
#4490=ORIENTED_EDGE('',*,*,#3271,.T.);
#4491=ORIENTED_EDGE('',*,*,#3220,.T.);
#4492=ORIENTED_EDGE('',*,*,#3236,.T.);
#4493=ORIENTED_EDGE('',*,*,#3279,.F.);
#4494=ORIENTED_EDGE('',*,*,#3318,.T.);
#4495=ORIENTED_EDGE('',*,*,#3304,.F.);
#4496=ORIENTED_EDGE('',*,*,#3318,.F.);
#4497=ORIENTED_EDGE('',*,*,#3224,.T.);
#4498=ORIENTED_EDGE('',*,*,#3225,.T.);
#4499=ORIENTED_EDGE('',*,*,#3222,.T.);
#4500=ORIENTED_EDGE('',*,*,#3223,.T.);
#4501=ORIENTED_EDGE('',*,*,#3240,.T.);
#4502=ORIENTED_EDGE('',*,*,#3241,.T.);
#4503=ORIENTED_EDGE('',*,*,#3238,.T.);
#4504=ORIENTED_EDGE('',*,*,#3239,.T.);
#4505=ORIENTED_EDGE('',*,*,#3305,.F.);
#4506=ORIENTED_EDGE('',*,*,#3319,.T.);
#4507=ORIENTED_EDGE('',*,*,#3280,.F.);
#4508=ORIENTED_EDGE('',*,*,#3319,.F.);
#4509=ORIENTED_EDGE('',*,*,#3216,.T.);
#4510=ORIENTED_EDGE('',*,*,#3217,.T.);
#4511=ORIENTED_EDGE('',*,*,#3214,.T.);
#4512=ORIENTED_EDGE('',*,*,#3215,.T.);
#4513=ORIENTED_EDGE('',*,*,#3232,.T.);
#4514=ORIENTED_EDGE('',*,*,#3233,.T.);
#4515=ORIENTED_EDGE('',*,*,#3230,.T.);
#4516=ORIENTED_EDGE('',*,*,#3231,.T.);
#4517=ORIENTED_EDGE('',*,*,#3306,.F.);
#4518=ORIENTED_EDGE('',*,*,#3320,.T.);
#4519=ORIENTED_EDGE('',*,*,#3281,.F.);
#4520=ORIENTED_EDGE('',*,*,#3320,.F.);
#4521=ORIENTED_EDGE('',*,*,#3289,.T.);
#4522=ORIENTED_EDGE('',*,*,#3307,.T.);
#4523=ORIENTED_EDGE('',*,*,#3274,.T.);
#4524=ORIENTED_EDGE('',*,*,#3321,.T.);
#4525=ORIENTED_EDGE('',*,*,#3321,.F.);
#4526=ORIENTED_EDGE('',*,*,#3273,.T.);
#4527=ORIENTED_EDGE('',*,*,#3322,.F.);
#4528=ORIENTED_EDGE('',*,*,#3290,.T.);
#4529=ORIENTED_EDGE('',*,*,#3272,.T.);
#4530=ORIENTED_EDGE('',*,*,#3317,.T.);
#4531=ORIENTED_EDGE('',*,*,#3291,.T.);
#4532=ORIENTED_EDGE('',*,*,#3322,.T.);
#4533=ORIENTED_EDGE('',*,*,#3260,.T.);
#4534=ORIENTED_EDGE('',*,*,#3255,.T.);
#4535=ORIENTED_EDGE('',*,*,#3303,.T.);
#4536=ORIENTED_EDGE('',*,*,#3323,.T.);
#4537=ORIENTED_EDGE('',*,*,#3323,.F.);
#4538=ORIENTED_EDGE('',*,*,#3302,.T.);
#4539=ORIENTED_EDGE('',*,*,#3324,.F.);
#4540=ORIENTED_EDGE('',*,*,#3261,.F.);
#4541=ORIENTED_EDGE('',*,*,#3301,.T.);
#4542=ORIENTED_EDGE('',*,*,#3312,.T.);
#4543=ORIENTED_EDGE('',*,*,#3262,.T.);
#4544=ORIENTED_EDGE('',*,*,#3324,.T.);
#4622=CYLINDRICAL_SURFACE('',#5758,2.5);
#4623=CYLINDRICAL_SURFACE('',#5760,2.5);
#4624=CYLINDRICAL_SURFACE('',#5762,2.5);
#4625=CYLINDRICAL_SURFACE('',#5764,2.5);
#4626=CYLINDRICAL_SURFACE('',#5766,2.5);
#4627=CYLINDRICAL_SURFACE('',#5768,2.5);
#4628=CYLINDRICAL_SURFACE('',#5770,2.5);
#4629=CYLINDRICAL_SURFACE('',#5772,2.5);
#4630=CYLINDRICAL_SURFACE('',#5800,10.5);
#4631=CYLINDRICAL_SURFACE('',#5801,10.5);
#4632=CYLINDRICAL_SURFACE('',#5802,17.5);
#4928=ADVANCED_FACE('',(#917),#4622,.F.);
#4929=ADVANCED_FACE('',(#918),#4623,.F.);
#4930=ADVANCED_FACE('',(#919),#4624,.F.);
#4931=ADVANCED_FACE('',(#920),#4625,.F.);
#4932=ADVANCED_FACE('',(#921),#4626,.F.);
#4933=ADVANCED_FACE('',(#922),#4627,.F.);
#4934=ADVANCED_FACE('',(#923),#4628,.F.);
#4935=ADVANCED_FACE('',(#924),#4629,.F.);
#4936=ADVANCED_FACE('',(#925),#596,.F.);
#4937=ADVANCED_FACE('',(#926),#597,.F.);
#4938=ADVANCED_FACE('',(#927),#598,.F.);
#4939=ADVANCED_FACE('',(#928,#460,#461),#599,.T.);
#4940=ADVANCED_FACE('',(#929),#600,.T.);
#4941=ADVANCED_FACE('',(#930,#462,#463,#464),#601,.T.);
#4942=ADVANCED_FACE('',(#931),#602,.T.);
#4943=ADVANCED_FACE('',(#932),#603,.T.);
#4944=ADVANCED_FACE('',(#933),#604,.T.);
#4945=ADVANCED_FACE('',(#934,#465,#466,#467),#605,.T.);
#4946=ADVANCED_FACE('',(#935,#468,#469),#606,.T.);
#4947=ADVANCED_FACE('',(#936),#607,.T.);
#4948=ADVANCED_FACE('',(#937),#608,.T.);
#4949=ADVANCED_FACE('',(#938),#609,.T.);
#4950=ADVANCED_FACE('',(#939,#470,#471),#610,.T.);
#4951=ADVANCED_FACE('',(#940),#611,.T.);
#4952=ADVANCED_FACE('',(#941),#612,.F.);
#4953=ADVANCED_FACE('',(#942),#613,.F.);
#4954=ADVANCED_FACE('',(#943),#614,.F.);
#4955=ADVANCED_FACE('',(#944,#472,#473),#615,.T.);
#4956=ADVANCED_FACE('',(#945,#474,#475,#476,#477),#4630,.F.);
#4957=ADVANCED_FACE('',(#946,#478,#479,#480,#481),#4631,.F.);
#4958=ADVANCED_FACE('',(#947),#4632,.F.);
#4959=ADVANCED_FACE('',(#948),#616,.T.);
#4960=ADVANCED_FACE('',(#949),#617,.T.);
#4961=ADVANCED_FACE('',(#950),#618,.T.);
#4962=ADVANCED_FACE('',(#951),#619,.T.);
#4963=ADVANCED_FACE('',(#952),#620,.T.);
#4964=ADVANCED_FACE('',(#953),#621,.T.);
#5021=CLOSED_SHELL('',(#4928,#4929,#4930,#4931,#4932,#4933,#4934,#4935,
#4936,#4937,#4938,#4939,#4940,#4941,#4942,#4943,#4944,#4945,#4946,#4947,
#4948,#4949,#4950,#4951,#4952,#4953,#4954,#4955,#4956,#4957,#4958,#4959,
#4960,#4961,#4962,#4963,#4964));
#5757=AXIS2_PLACEMENT_3D('',#8957,#7250,#7251);
#5758=AXIS2_PLACEMENT_3D('',#8958,#7252,#7253);
#5759=AXIS2_PLACEMENT_3D('',#8960,#7254,#7255);
#5760=AXIS2_PLACEMENT_3D('',#9000,#7257,#7258);
#5761=AXIS2_PLACEMENT_3D('',#9041,#7260,#7261);
#5762=AXIS2_PLACEMENT_3D('',#9042,#7262,#7263);
#5763=AXIS2_PLACEMENT_3D('',#9044,#7264,#7265);
#5764=AXIS2_PLACEMENT_3D('',#9084,#7267,#7268);
#5765=AXIS2_PLACEMENT_3D('',#9125,#7270,#7271);
#5766=AXIS2_PLACEMENT_3D('',#9126,#7272,#7273);
#5767=AXIS2_PLACEMENT_3D('',#9128,#7274,#7275);
#5768=AXIS2_PLACEMENT_3D('',#9168,#7277,#7278);
#5769=AXIS2_PLACEMENT_3D('',#9209,#7280,#7281);
#5770=AXIS2_PLACEMENT_3D('',#9210,#7282,#7283);
#5771=AXIS2_PLACEMENT_3D('',#9212,#7284,#7285);
#5772=AXIS2_PLACEMENT_3D('',#9252,#7287,#7288);
#5773=AXIS2_PLACEMENT_3D('',#9293,#7290,#7291);
#5774=AXIS2_PLACEMENT_3D('',#9294,#7292,#7293);
#5775=AXIS2_PLACEMENT_3D('',#9303,#7298,#7299);
#5776=AXIS2_PLACEMENT_3D('',#9309,#7303,#7304);
#5777=AXIS2_PLACEMENT_3D('',#9315,#7308,#7309);
#5778=AXIS2_PLACEMENT_3D('',#9321,#7313,#7314);
#5779=AXIS2_PLACEMENT_3D('',#9327,#7318,#7319);
#5780=AXIS2_PLACEMENT_3D('',#9366,#7339,#7340);
#5781=AXIS2_PLACEMENT_3D('',#9368,#7341,#7342);
#5782=AXIS2_PLACEMENT_3D('',#9370,#7343,#7344);
#5783=AXIS2_PLACEMENT_3D('',#9371,#7345,#7346);
#5784=AXIS2_PLACEMENT_3D('',#9377,#7350,#7351);
#5785=AXIS2_PLACEMENT_3D('',#9381,#7354,#7355);
#5786=AXIS2_PLACEMENT_3D('',#9383,#7357,#7358);
#5787=AXIS2_PLACEMENT_3D('',#9416,#7375,#7376);
#5788=AXIS2_PLACEMENT_3D('',#9418,#7377,#7378);
#5789=AXIS2_PLACEMENT_3D('',#9420,#7379,#7380);
#5790=AXIS2_PLACEMENT_3D('',#9421,#7381,#7382);
#5791=AXIS2_PLACEMENT_3D('',#9423,#7384,#7385);
#5792=AXIS2_PLACEMENT_3D('',#9426,#7388,#7389);
#5793=AXIS2_PLACEMENT_3D('',#9428,#7391,#7392);
#5794=AXIS2_PLACEMENT_3D('',#9430,#7394,#7395);
#5795=AXIS2_PLACEMENT_3D('',#9432,#7397,#7398);
#5796=AXIS2_PLACEMENT_3D('',#9434,#7400,#7401);
#5797=AXIS2_PLACEMENT_3D('',#9437,#7404,#7405);
#5798=AXIS2_PLACEMENT_3D('',#9439,#7407,#7408);
#5799=AXIS2_PLACEMENT_3D('',#9440,#7409,#7410);
#5800=AXIS2_PLACEMENT_3D('',#9442,#7412,#7413);
#5801=AXIS2_PLACEMENT_3D('',#9444,#7415,#7416);
#5802=AXIS2_PLACEMENT_3D('',#9446,#7418,#7419);
#5803=AXIS2_PLACEMENT_3D('',#9448,#7421,#7422);
#5804=AXIS2_PLACEMENT_3D('',#9450,#7424,#7425);
#5805=AXIS2_PLACEMENT_3D('',#9452,#7427,#7428);
#5806=AXIS2_PLACEMENT_3D('',#9453,#7429,#7430);
#5807=AXIS2_PLACEMENT_3D('',#9455,#7432,#7433);
#5808=AXIS2_PLACEMENT_3D('',#9457,#7435,#7436);
#7250=DIRECTION('axis',(0.,0.,1.));
#7251=DIRECTION('refdir',(1.,0.,0.));
#7252=DIRECTION('center_axis',(0.,0.,-1.));
#7253=DIRECTION('ref_axis',(-1.,0.,0.));
#7254=DIRECTION('center_axis',(0.,0.,-1.));
#7255=DIRECTION('ref_axis',(-1.,0.,0.));
#7256=DIRECTION('',(0.,0.,-1.));
#7257=DIRECTION('center_axis',(0.,0.,-1.));
#7258=DIRECTION('ref_axis',(-1.,0.,0.));
#7259=DIRECTION('',(0.,0.,-1.));
#7260=DIRECTION('center_axis',(0.,0.,1.));
#7261=DIRECTION('ref_axis',(-1.,0.,0.));
#7262=DIRECTION('center_axis',(0.,0.,-1.));
#7263=DIRECTION('ref_axis',(-1.,0.,0.));
#7264=DIRECTION('center_axis',(0.,0.,-1.));
#7265=DIRECTION('ref_axis',(-1.,0.,0.));
#7266=DIRECTION('',(0.,0.,-1.));
#7267=DIRECTION('center_axis',(0.,0.,-1.));
#7268=DIRECTION('ref_axis',(-1.,0.,0.));
#7269=DIRECTION('',(0.,0.,-1.));
#7270=DIRECTION('center_axis',(0.,0.,1.));
#7271=DIRECTION('ref_axis',(-1.,0.,0.));
#7272=DIRECTION('center_axis',(0.,0.,-1.));
#7273=DIRECTION('ref_axis',(-1.,0.,0.));
#7274=DIRECTION('center_axis',(0.,0.,-1.));
#7275=DIRECTION('ref_axis',(-1.,0.,0.));
#7276=DIRECTION('',(0.,0.,-1.));
#7277=DIRECTION('center_axis',(0.,0.,-1.));
#7278=DIRECTION('ref_axis',(-1.,0.,0.));
#7279=DIRECTION('',(0.,0.,-1.));
#7280=DIRECTION('center_axis',(0.,0.,1.));
#7281=DIRECTION('ref_axis',(-1.,0.,0.));
#7282=DIRECTION('center_axis',(0.,0.,-1.));
#7283=DIRECTION('ref_axis',(-1.,0.,0.));
#7284=DIRECTION('center_axis',(0.,0.,-1.));
#7285=DIRECTION('ref_axis',(-1.,0.,0.));
#7286=DIRECTION('',(0.,0.,-1.));
#7287=DIRECTION('center_axis',(0.,0.,-1.));
#7288=DIRECTION('ref_axis',(-1.,0.,0.));
#7289=DIRECTION('',(0.,0.,-1.));
#7290=DIRECTION('center_axis',(0.,0.,1.));
#7291=DIRECTION('ref_axis',(-1.,0.,0.));
#7292=DIRECTION('center_axis',(0.,-0.707106781186547,0.707106781186548));
#7293=DIRECTION('ref_axis',(0.,-0.707106781186548,-0.707106781186547));
#7294=DIRECTION('',(0.,-0.707106781186548,-0.707106781186547));
#7295=DIRECTION('',(1.,0.,0.));
#7296=DIRECTION('',(0.,0.707106781186548,0.707106781186547));
#7297=DIRECTION('',(1.,0.,0.));
#7298=DIRECTION('center_axis',(0.,0.,1.));
#7299=DIRECTION('ref_axis',(0.,-1.,0.));
#7300=DIRECTION('',(0.,-1.,0.));
#7301=DIRECTION('',(1.,0.,0.));
#7302=DIRECTION('',(0.,1.,0.));
#7303=DIRECTION('center_axis',(0.,0.707106781186548,0.707106781186548));
#7304=DIRECTION('ref_axis',(0.,-0.707106781186548,0.707106781186548));
#7305=DIRECTION('',(0.,-0.707106781186547,0.707106781186547));
#7306=DIRECTION('',(-1.,0.,0.));
#7307=DIRECTION('',(0.,0.707106781186547,-0.707106781186547));
#7308=DIRECTION('center_axis',(0.,0.,-1.));
#7309=DIRECTION('ref_axis',(-1.,0.,0.));
#7310=DIRECTION('',(0.,-1.,0.));
#7311=DIRECTION('',(1.,0.,0.));
#7312=DIRECTION('',(0.,1.,0.));
#7313=DIRECTION('center_axis',(0.,0.,-1.));
#7314=DIRECTION('ref_axis',(-1.,0.,0.));
#7315=DIRECTION('',(0.,1.,0.));
#7316=DIRECTION('',(1.,0.,0.));
#7317=DIRECTION('',(0.,-1.,0.));
#7318=DIRECTION('center_axis',(-1.,0.,0.));
#7319=DIRECTION('ref_axis',(0.,-1.,0.));
#7320=DIRECTION('',(0.,0.707106781186547,-0.707106781186548));
#7321=DIRECTION('',(0.,0.,1.));
#7322=DIRECTION('',(0.,-0.707106781186547,-0.707106781186548));
#7323=DIRECTION('',(0.,-1.,0.));
#7324=DIRECTION('',(0.,0.707106781186548,-0.707106781186547));
#7325=DIRECTION('',(0.,1.,0.));
#7326=DIRECTION('',(0.,0.707106781186547,0.707106781186547));
#7327=DIRECTION('',(0.,-1.,0.));
#7328=DIRECTION('',(0.,0.707106781186547,-0.707106781186547));
#7329=DIRECTION('',(0.,1.,0.));
#7330=DIRECTION('',(0.,0.707106781186548,0.707106781186547));
#7331=DIRECTION('',(0.,-1.,0.));
#7332=DIRECTION('',(0.,-0.707106781186547,0.707106781186548));
#7333=DIRECTION('',(0.,0.,1.));
#7334=DIRECTION('',(0.,0.707106781186547,0.707106781186548));
#7335=DIRECTION('',(0.,1.,0.));
#7336=DIRECTION('',(0.,-0.707106781186548,0.707106781186547));
#7337=DIRECTION('',(0.,-1.,0.));
#7338=DIRECTION('',(0.,-0.707106781186547,-0.707106781186547));
#7339=DIRECTION('center_axis',(1.,0.,0.));
#7340=DIRECTION('ref_axis',(0.,-1.,0.));
#7341=DIRECTION('center_axis',(1.,0.,0.));
#7342=DIRECTION('ref_axis',(0.,1.,0.));
#7343=DIRECTION('center_axis',(1.,0.,0.));
#7344=DIRECTION('ref_axis',(0.,1.,0.));
#7345=DIRECTION('center_axis',(0.,-0.707106781186547,-0.707106781186548));
#7346=DIRECTION('ref_axis',(0.,0.707106781186548,-0.707106781186547));
#7347=DIRECTION('',(-1.,0.,0.));
#7348=DIRECTION('',(0.,0.707106781186548,-0.707106781186547));
#7349=DIRECTION('',(1.,0.,0.));
#7350=DIRECTION('center_axis',(0.,0.,-1.));
#7351=DIRECTION('ref_axis',(0.,1.,0.));
#7352=DIRECTION('',(0.,1.,0.));
#7353=DIRECTION('',(1.,0.,0.));
#7354=DIRECTION('center_axis',(0.,0.707106781186548,-0.707106781186548));
#7355=DIRECTION('ref_axis',(0.,0.707106781186548,0.707106781186548));
#7356=DIRECTION('',(0.,0.707106781186547,0.707106781186547));
#7357=DIRECTION('center_axis',(1.,0.,0.));
#7358=DIRECTION('ref_axis',(0.,1.,0.));
#7359=DIRECTION('',(0.,-1.,0.));
#7360=DIRECTION('',(0.,-0.707106781186547,-0.707106781186548));
#7361=DIRECTION('',(0.,0.,-1.));
#7362=DIRECTION('',(0.,0.707106781186547,-0.707106781186548));
#7363=DIRECTION('',(0.,1.,0.));
#7364=DIRECTION('',(0.,-0.707106781186548,-0.707106781186547));
#7365=DIRECTION('',(0.,-1.,0.));
#7366=DIRECTION('',(0.,-0.707106781186547,0.707106781186547));
#7367=DIRECTION('',(0.,1.,0.));
#7368=DIRECTION('',(0.,-0.707106781186547,-0.707106781186547));
#7369=DIRECTION('',(0.,-1.,0.));
#7370=DIRECTION('',(0.,-0.707106781186548,0.707106781186547));
#7371=DIRECTION('',(0.,1.,0.));
#7372=DIRECTION('',(0.,0.707106781186547,0.707106781186548));
#7373=DIRECTION('',(0.,0.,1.));
#7374=DIRECTION('',(0.,-0.707106781186547,0.707106781186548));
#7375=DIRECTION('center_axis',(-1.,0.,0.));
#7376=DIRECTION('ref_axis',(0.,-1.,0.));
#7377=DIRECTION('center_axis',(-1.,0.,0.));
#7378=DIRECTION('ref_axis',(0.,1.,0.));
#7379=DIRECTION('center_axis',(-1.,0.,0.));
#7380=DIRECTION('ref_axis',(0.,1.,0.));
#7381=DIRECTION('center_axis',(0.,0.,-1.));
#7382=DIRECTION('ref_axis',(-1.,0.,0.));
#7383=DIRECTION('',(-1.,0.,0.));
#7384=DIRECTION('center_axis',(0.,0.707106781186547,0.707106781186548));
#7385=DIRECTION('ref_axis',(0.,-0.707106781186548,0.707106781186547));
#7386=DIRECTION('',(-1.,0.,0.));
#7387=DIRECTION('',(1.,0.,0.));
#7388=DIRECTION('center_axis',(0.,0.,1.));
#7389=DIRECTION('ref_axis',(0.,-1.,0.));
#7390=DIRECTION('',(1.,0.,0.));
#7391=DIRECTION('center_axis',(0.,-0.707106781186548,0.707106781186548));
#7392=DIRECTION('ref_axis',(0.,-0.707106781186548,-0.707106781186548));
#7393=DIRECTION('',(1.,0.,0.));
#7394=DIRECTION('center_axis',(0.,0.,1.));
#7395=DIRECTION('ref_axis',(1.,0.,0.));
#7396=DIRECTION('',(-1.,0.,0.));
#7397=DIRECTION('center_axis',(0.,0.,1.));
#7398=DIRECTION('ref_axis',(1.,0.,0.));
#7399=DIRECTION('',(-1.,0.,0.));
#7400=DIRECTION('center_axis',(0.,0.707106781186547,-0.707106781186548));
#7401=DIRECTION('ref_axis',(0.,0.707106781186548,0.707106781186547));
#7402=DIRECTION('',(1.,0.,0.));
#7403=DIRECTION('',(1.,0.,0.));
#7404=DIRECTION('center_axis',(0.,0.,-1.));
#7405=DIRECTION('ref_axis',(0.,1.,0.));
#7406=DIRECTION('',(1.,0.,0.));
#7407=DIRECTION('center_axis',(0.,-0.707106781186548,-0.707106781186548));
#7408=DIRECTION('ref_axis',(0.,0.707106781186548,-0.707106781186548));
#7409=DIRECTION('center_axis',(0.,0.,1.));
#7410=DIRECTION('ref_axis',(1.,0.,0.));
#7411=DIRECTION('',(1.,0.,0.));
#7412=DIRECTION('center_axis',(1.,0.,0.));
#7413=DIRECTION('ref_axis',(0.,-1.,0.));
#7414=DIRECTION('',(1.,0.,0.));
#7415=DIRECTION('center_axis',(-1.,0.,0.));
#7416=DIRECTION('ref_axis',(0.,1.,0.));
#7417=DIRECTION('',(-1.,0.,0.));
#7418=DIRECTION('center_axis',(-1.,0.,0.));
#7419=DIRECTION('ref_axis',(0.,1.,0.));
#7420=DIRECTION('',(-1.,0.,0.));
#7421=DIRECTION('center_axis',(0.,0.707106781186548,-0.707106781186547));
#7422=DIRECTION('ref_axis',(-1.,0.,0.));
#7423=DIRECTION('',(1.,0.,0.));
#7424=DIRECTION('center_axis',(0.,1.,0.));
#7425=DIRECTION('ref_axis',(-1.,0.,0.));
#7426=DIRECTION('',(-1.,0.,0.));
#7427=DIRECTION('center_axis',(0.,0.707106781186548,0.707106781186547));
#7428=DIRECTION('ref_axis',(1.,0.,0.));
#7429=DIRECTION('center_axis',(0.,-0.707106781186548,-0.707106781186547));
#7430=DIRECTION('ref_axis',(-1.,0.,0.));
#7431=DIRECTION('',(-1.,0.,0.));
#7432=DIRECTION('center_axis',(0.,-1.,0.));
#7433=DIRECTION('ref_axis',(1.,0.,0.));
#7434=DIRECTION('',(1.,0.,0.));
#7435=DIRECTION('center_axis',(0.,-0.707106781186548,0.707106781186547));
#7436=DIRECTION('ref_axis',(1.,0.,0.));
#8957=CARTESIAN_POINT('',(0.,0.,0.));
#8958=CARTESIAN_POINT('Origin',(-28.795061332806,-41.6915321010441,20.));
#8959=CARTESIAN_POINT('',(-26.295061332806,-41.6915321010441,20.));
#8960=CARTESIAN_POINT('Origin',(-28.795061332806,-41.6915321010441,20.));
#8961=CARTESIAN_POINT('',(-26.295061332806,-41.6915321010441,1.76587979759228));
#8962=CARTESIAN_POINT('',(-26.295061332806,-41.6915321010441,20.));
#8963=CARTESIAN_POINT('',(-28.795061332806,-44.1915321010441,0.356833582029305));
#8964=CARTESIAN_POINT('Ctrl Pts',(-28.795061332806,-44.1915321010441,0.356833582029284));
#8965=CARTESIAN_POINT('Ctrl Pts',(-28.477785430142,-44.1915321010441,0.356833582029284));
#8966=CARTESIAN_POINT('Ctrl Pts',(-28.1469294547233,-44.1275251245074,0.406497032324426));
#8967=CARTESIAN_POINT('Ctrl Pts',(-27.5495967417843,-43.8830970093849,0.584048414544644));
#8968=CARTESIAN_POINT('Ctrl Pts',(-27.2824224552858,-43.7030327750914,0.710075190333896));
#8969=CARTESIAN_POINT('Ctrl Pts',(-26.8364104627744,-43.2788343380328,0.982143846508312));
#8970=CARTESIAN_POINT('Ctrl Pts',(-26.634884040132,-42.9955925725868,1.15080480840549));
#8971=CARTESIAN_POINT('Ctrl Pts',(-26.3640331527432,-42.3675807949546,1.47762784261656));
#8972=CARTESIAN_POINT('Ctrl Pts',(-26.295061332806,-42.0223600026362,1.63521545889971));
#8973=CARTESIAN_POINT('Ctrl Pts',(-26.295061332806,-41.6915321010441,1.76587979759228));
#8974=CARTESIAN_POINT('Ctrl Pts',(-26.295061332806,-41.6915321010441,1.76587979759228));
#8975=CARTESIAN_POINT('Ctrl Pts',(-26.295061332806,-41.3866319916517,1.88630365231953));
#8976=CARTESIAN_POINT('Ctrl Pts',(-26.3545217120232,-41.0538505476253,1.99948444500592));
#8977=CARTESIAN_POINT('Ctrl Pts',(-26.6094575005743,-40.432164168516,2.17871269254273));
#8978=CARTESIAN_POINT('Ctrl Pts',(-26.8052572776176,-40.14362590236,2.24556937536941));
#8979=CARTESIAN_POINT('Ctrl Pts',(-27.2559905957869,-39.697227181252,2.33582555282254));
#8980=CARTESIAN_POINT('Ctrl Pts',(-27.5353468960521,-39.5067960121042,2.36674372859812));
#8981=CARTESIAN_POINT('Ctrl Pts',(-28.1484345319317,-39.2539459288562,2.40438278535118));
#8982=CARTESIAN_POINT('Ctrl Pts',(-28.4821173645511,-39.1915321010441,2.41192340176922));
#8983=CARTESIAN_POINT('Ctrl Pts',(-29.1080053010609,-39.1915321010441,2.41192340176922));
#8984=CARTESIAN_POINT('Ctrl Pts',(-29.4416881336803,-39.2539459288562,2.40438278535118));
#8985=CARTESIAN_POINT('Ctrl Pts',(-30.0547757695599,-39.5067960121042,2.36674372859812));
#8986=CARTESIAN_POINT('Ctrl Pts',(-30.3341320698251,-39.697227181252,2.33582555282254));
#8987=CARTESIAN_POINT('Ctrl Pts',(-30.7848653879944,-40.14362590236,2.24556937536941));
#8988=CARTESIAN_POINT('Ctrl Pts',(-30.9806651650377,-40.432164168516,2.17871269254273));
#8989=CARTESIAN_POINT('Ctrl Pts',(-31.2356009535887,-41.0538505476253,1.99948444500592));
#8990=CARTESIAN_POINT('Ctrl Pts',(-31.295061332806,-41.3866319916517,1.88630365231953));
#8991=CARTESIAN_POINT('Ctrl Pts',(-31.295061332806,-42.0223600026362,1.63521545889971));
#8992=CARTESIAN_POINT('Ctrl Pts',(-31.2260895128688,-42.3675807949547,1.47762784261656));
#8993=CARTESIAN_POINT('Ctrl Pts',(-30.95523862548,-42.9955925725868,1.15080480840548));
#8994=CARTESIAN_POINT('Ctrl Pts',(-30.7537122028376,-43.2788343380328,0.982143846508312));
#8995=CARTESIAN_POINT('Ctrl Pts',(-30.3077002103262,-43.7030327750914,0.710075190333895));
#8996=CARTESIAN_POINT('Ctrl Pts',(-30.0405259238277,-43.8830970093849,0.584048414544644));
#8997=CARTESIAN_POINT('Ctrl Pts',(-29.4431932108887,-44.1275251245074,0.406497032324426));
#8998=CARTESIAN_POINT('Ctrl Pts',(-29.11233723547,-44.1915321010441,0.356833582029284));
#8999=CARTESIAN_POINT('Ctrl Pts',(-28.795061332806,-44.1915321010441,0.356833582029284));
#9000=CARTESIAN_POINT('Origin',(-28.795061332806,-41.6915321010441,20.));
#9001=CARTESIAN_POINT('',(-28.795061332806,-44.1915321010441,-16.3568335820293));
#9002=CARTESIAN_POINT('',(-26.295061332806,-41.6915321010441,-17.7658797975923));
#9003=CARTESIAN_POINT('Ctrl Pts',(-28.795061332806,-44.1915321010441,-16.3568335820293));
#9004=CARTESIAN_POINT('Ctrl Pts',(-29.1123372354701,-44.1915321010441,-16.3568335820293));
#9005=CARTESIAN_POINT('Ctrl Pts',(-29.4431932108887,-44.1275251245074,-16.4064970323244));
#9006=CARTESIAN_POINT('Ctrl Pts',(-30.0405259238277,-43.8830970093849,-16.5840484145446));
#9007=CARTESIAN_POINT('Ctrl Pts',(-30.3077002103262,-43.7030327750914,-16.7100751903339));
#9008=CARTESIAN_POINT('Ctrl Pts',(-30.7537122028376,-43.2788343380328,-16.9821438465083));
#9009=CARTESIAN_POINT('Ctrl Pts',(-30.95523862548,-42.9955925725868,-17.1508048084055));
#9010=CARTESIAN_POINT('Ctrl Pts',(-31.2260895128688,-42.3675807949546,-17.4776278426165));
#9011=CARTESIAN_POINT('Ctrl Pts',(-31.295061332806,-42.0223600026362,-17.6352154588997));
#9012=CARTESIAN_POINT('Ctrl Pts',(-31.295061332806,-41.3866319916517,-17.8863036523195));
#9013=CARTESIAN_POINT('Ctrl Pts',(-31.2356009535887,-41.0538505476253,-17.9994844450059));
#9014=CARTESIAN_POINT('Ctrl Pts',(-30.9806651650377,-40.432164168516,-18.1787126925427));
#9015=CARTESIAN_POINT('Ctrl Pts',(-30.7848653879944,-40.14362590236,-18.2455693753694));
#9016=CARTESIAN_POINT('Ctrl Pts',(-30.3341320698251,-39.697227181252,-18.3358255528225));
#9017=CARTESIAN_POINT('Ctrl Pts',(-30.0547757695599,-39.5067960121042,-18.3667437285981));
#9018=CARTESIAN_POINT('Ctrl Pts',(-29.4416881336803,-39.2539459288562,-18.4043827853512));
#9019=CARTESIAN_POINT('Ctrl Pts',(-29.1080053010609,-39.1915321010441,-18.4119234017692));
#9020=CARTESIAN_POINT('Ctrl Pts',(-28.4821173645511,-39.1915321010441,-18.4119234017692));
#9021=CARTESIAN_POINT('Ctrl Pts',(-28.1484345319317,-39.2539459288562,-18.4043827853512));
#9022=CARTESIAN_POINT('Ctrl Pts',(-27.5353468960521,-39.5067960121042,-18.3667437285981));
#9023=CARTESIAN_POINT('Ctrl Pts',(-27.2559905957869,-39.697227181252,-18.3358255528225));
#9024=CARTESIAN_POINT('Ctrl Pts',(-26.8052572776176,-40.14362590236,-18.2455693753694));
#9025=CARTESIAN_POINT('Ctrl Pts',(-26.6094575005743,-40.432164168516,-18.1787126925427));
#9026=CARTESIAN_POINT('Ctrl Pts',(-26.3545217120232,-41.0538505476253,-17.9994844450059));
#9027=CARTESIAN_POINT('Ctrl Pts',(-26.295061332806,-41.3866319916517,-17.8863036523195));
#9028=CARTESIAN_POINT('Ctrl Pts',(-26.295061332806,-41.6915321010441,-17.7658797975923));
#9029=CARTESIAN_POINT('Ctrl Pts',(-26.295061332806,-41.6915321010441,-17.7658797975923));
#9030=CARTESIAN_POINT('Ctrl Pts',(-26.295061332806,-42.0223600026362,-17.6352154588997));
#9031=CARTESIAN_POINT('Ctrl Pts',(-26.3640331527432,-42.3675807949547,-17.4776278426165));
#9032=CARTESIAN_POINT('Ctrl Pts',(-26.634884040132,-42.9955925725868,-17.1508048084055));
#9033=CARTESIAN_POINT('Ctrl Pts',(-26.8364104627744,-43.2788343380328,-16.9821438465083));
#9034=CARTESIAN_POINT('Ctrl Pts',(-27.2824224552858,-43.7030327750914,-16.7100751903339));
#9035=CARTESIAN_POINT('Ctrl Pts',(-27.5495967417843,-43.8830970093849,-16.5840484145446));
#9036=CARTESIAN_POINT('Ctrl Pts',(-28.1469294547233,-44.1275251245074,-16.4064970323244));
#9037=CARTESIAN_POINT('Ctrl Pts',(-28.477785430142,-44.1915321010441,-16.3568335820293));
#9038=CARTESIAN_POINT('Ctrl Pts',(-28.795061332806,-44.1915321010441,-16.3568335820293));
#9039=CARTESIAN_POINT('',(-26.295061332806,-41.6915321010441,-20.));
#9040=CARTESIAN_POINT('',(-26.295061332806,-41.6915321010441,20.));
#9041=CARTESIAN_POINT('Origin',(-28.795061332806,-41.6915321010441,-20.));
#9042=CARTESIAN_POINT('Origin',(28.795061332806,41.6915321010441,20.));
#9043=CARTESIAN_POINT('',(31.295061332806,41.6915321010441,20.));
#9044=CARTESIAN_POINT('Origin',(28.795061332806,41.6915321010441,20.));
#9045=CARTESIAN_POINT('',(31.295061332806,41.6915321010441,1.76587979759228));
#9046=CARTESIAN_POINT('',(31.295061332806,41.6915321010441,20.));
#9047=CARTESIAN_POINT('',(28.795061332806,44.1915321010441,0.356833582029305));
#9048=CARTESIAN_POINT('Ctrl Pts',(28.795061332806,44.1915321010441,0.356833582029284));
#9049=CARTESIAN_POINT('Ctrl Pts',(28.477785430142,44.1915321010441,0.356833582029284));
#9050=CARTESIAN_POINT('Ctrl Pts',(28.1469294547233,44.1275251245074,0.406497032324426));
#9051=CARTESIAN_POINT('Ctrl Pts',(27.5495967417843,43.8830970093849,0.584048414544644));
#9052=CARTESIAN_POINT('Ctrl Pts',(27.2824224552858,43.7030327750914,0.710075190333896));
#9053=CARTESIAN_POINT('Ctrl Pts',(26.8364104627744,43.2788343380328,0.982143846508312));
#9054=CARTESIAN_POINT('Ctrl Pts',(26.634884040132,42.9955925725868,1.15080480840549));
#9055=CARTESIAN_POINT('Ctrl Pts',(26.3640331527432,42.3675807949546,1.47762784261656));
#9056=CARTESIAN_POINT('Ctrl Pts',(26.295061332806,42.0223600026362,1.63521545889971));
#9057=CARTESIAN_POINT('Ctrl Pts',(26.295061332806,41.3866319916517,1.88630365231953));
#9058=CARTESIAN_POINT('Ctrl Pts',(26.3545217120232,41.0538505476253,1.99948444500592));
#9059=CARTESIAN_POINT('Ctrl Pts',(26.6094575005743,40.432164168516,2.17871269254273));
#9060=CARTESIAN_POINT('Ctrl Pts',(26.8052572776176,40.14362590236,2.24556937536941));
#9061=CARTESIAN_POINT('Ctrl Pts',(27.2559905957869,39.697227181252,2.33582555282254));
#9062=CARTESIAN_POINT('Ctrl Pts',(27.5353468960521,39.5067960121042,2.36674372859812));
#9063=CARTESIAN_POINT('Ctrl Pts',(28.1484345319317,39.2539459288562,2.40438278535118));
#9064=CARTESIAN_POINT('Ctrl Pts',(28.4821173645511,39.1915321010441,2.41192340176922));
#9065=CARTESIAN_POINT('Ctrl Pts',(29.1080053010609,39.1915321010441,2.41192340176922));
#9066=CARTESIAN_POINT('Ctrl Pts',(29.4416881336803,39.2539459288562,2.40438278535118));
#9067=CARTESIAN_POINT('Ctrl Pts',(30.0547757695599,39.5067960121042,2.36674372859812));
#9068=CARTESIAN_POINT('Ctrl Pts',(30.3341320698251,39.697227181252,2.33582555282254));
#9069=CARTESIAN_POINT('Ctrl Pts',(30.7848653879944,40.14362590236,2.24556937536941));
#9070=CARTESIAN_POINT('Ctrl Pts',(30.9806651650377,40.432164168516,2.17871269254273));
#9071=CARTESIAN_POINT('Ctrl Pts',(31.2356009535887,41.0538505476253,1.99948444500592));
#9072=CARTESIAN_POINT('Ctrl Pts',(31.295061332806,41.3866319916517,1.88630365231953));
#9073=CARTESIAN_POINT('Ctrl Pts',(31.295061332806,41.6915321010441,1.76587979759227));
#9074=CARTESIAN_POINT('Ctrl Pts',(31.295061332806,41.6915321010441,1.76587979759227));
#9075=CARTESIAN_POINT('Ctrl Pts',(31.295061332806,42.0223600026362,1.63521545889971));
#9076=CARTESIAN_POINT('Ctrl Pts',(31.2260895128688,42.3675807949547,1.47762784261656));
#9077=CARTESIAN_POINT('Ctrl Pts',(30.95523862548,42.9955925725868,1.15080480840548));
#9078=CARTESIAN_POINT('Ctrl Pts',(30.7537122028376,43.2788343380328,0.982143846508312));
#9079=CARTESIAN_POINT('Ctrl Pts',(30.3077002103262,43.7030327750914,0.710075190333895));
#9080=CARTESIAN_POINT('Ctrl Pts',(30.0405259238277,43.8830970093849,0.584048414544644));
#9081=CARTESIAN_POINT('Ctrl Pts',(29.4431932108887,44.1275251245074,0.406497032324426));
#9082=CARTESIAN_POINT('Ctrl Pts',(29.11233723547,44.1915321010441,0.356833582029284));
#9083=CARTESIAN_POINT('Ctrl Pts',(28.795061332806,44.1915321010441,0.356833582029284));
#9084=CARTESIAN_POINT('Origin',(28.795061332806,41.6915321010441,20.));
#9085=CARTESIAN_POINT('',(28.795061332806,44.1915321010441,-16.3568335820293));
#9086=CARTESIAN_POINT('',(31.295061332806,41.6915321010441,-17.7658797975923));
#9087=CARTESIAN_POINT('Ctrl Pts',(28.795061332806,44.1915321010441,-16.3568335820293));
#9088=CARTESIAN_POINT('Ctrl Pts',(29.1123372354701,44.1915321010441,-16.3568335820293));
#9089=CARTESIAN_POINT('Ctrl Pts',(29.4431932108887,44.1275251245074,-16.4064970323244));
#9090=CARTESIAN_POINT('Ctrl Pts',(30.0405259238277,43.8830970093849,-16.5840484145446));
#9091=CARTESIAN_POINT('Ctrl Pts',(30.3077002103262,43.7030327750914,-16.7100751903339));
#9092=CARTESIAN_POINT('Ctrl Pts',(30.7537122028376,43.2788343380328,-16.9821438465083));
#9093=CARTESIAN_POINT('Ctrl Pts',(30.95523862548,42.9955925725868,-17.1508048084055));
#9094=CARTESIAN_POINT('Ctrl Pts',(31.2260895128688,42.3675807949546,-17.4776278426165));
#9095=CARTESIAN_POINT('Ctrl Pts',(31.295061332806,42.0223600026362,-17.6352154588997));
#9096=CARTESIAN_POINT('Ctrl Pts',(31.295061332806,41.6915321010441,-17.7658797975923));
#9097=CARTESIAN_POINT('Ctrl Pts',(31.295061332806,41.6915321010441,-17.7658797975923));
#9098=CARTESIAN_POINT('Ctrl Pts',(31.295061332806,41.3866319916517,-17.8863036523195));
#9099=CARTESIAN_POINT('Ctrl Pts',(31.2356009535887,41.0538505476253,-17.9994844450059));
#9100=CARTESIAN_POINT('Ctrl Pts',(30.9806651650377,40.432164168516,-18.1787126925427));
#9101=CARTESIAN_POINT('Ctrl Pts',(30.7848653879944,40.14362590236,-18.2455693753694));
#9102=CARTESIAN_POINT('Ctrl Pts',(30.3341320698251,39.697227181252,-18.3358255528225));
#9103=CARTESIAN_POINT('Ctrl Pts',(30.0547757695599,39.5067960121042,-18.3667437285981));
#9104=CARTESIAN_POINT('Ctrl Pts',(29.4416881336803,39.2539459288562,-18.4043827853512));
#9105=CARTESIAN_POINT('Ctrl Pts',(29.1080053010609,39.1915321010441,-18.4119234017692));
#9106=CARTESIAN_POINT('Ctrl Pts',(28.4821173645511,39.1915321010441,-18.4119234017692));
#9107=CARTESIAN_POINT('Ctrl Pts',(28.1484345319317,39.2539459288562,-18.4043827853512));
#9108=CARTESIAN_POINT('Ctrl Pts',(27.5353468960521,39.5067960121042,-18.3667437285981));
#9109=CARTESIAN_POINT('Ctrl Pts',(27.2559905957869,39.697227181252,-18.3358255528225));
#9110=CARTESIAN_POINT('Ctrl Pts',(26.8052572776176,40.14362590236,-18.2455693753694));
#9111=CARTESIAN_POINT('Ctrl Pts',(26.6094575005743,40.432164168516,-18.1787126925427));
#9112=CARTESIAN_POINT('Ctrl Pts',(26.3545217120232,41.0538505476253,-17.9994844450059));
#9113=CARTESIAN_POINT('Ctrl Pts',(26.295061332806,41.3866319916517,-17.8863036523195));
#9114=CARTESIAN_POINT('Ctrl Pts',(26.295061332806,42.0223600026362,-17.6352154588997));
#9115=CARTESIAN_POINT('Ctrl Pts',(26.3640331527432,42.3675807949547,-17.4776278426165));
#9116=CARTESIAN_POINT('Ctrl Pts',(26.634884040132,42.9955925725868,-17.1508048084055));
#9117=CARTESIAN_POINT('Ctrl Pts',(26.8364104627744,43.2788343380328,-16.9821438465083));
#9118=CARTESIAN_POINT('Ctrl Pts',(27.2824224552858,43.7030327750914,-16.7100751903339));
#9119=CARTESIAN_POINT('Ctrl Pts',(27.5495967417843,43.8830970093849,-16.5840484145446));
#9120=CARTESIAN_POINT('Ctrl Pts',(28.1469294547233,44.1275251245074,-16.4064970323244));
#9121=CARTESIAN_POINT('Ctrl Pts',(28.477785430142,44.1915321010441,-16.3568335820293));
#9122=CARTESIAN_POINT('Ctrl Pts',(28.795061332806,44.1915321010441,-16.3568335820293));
#9123=CARTESIAN_POINT('',(31.295061332806,41.6915321010441,-20.));
#9124=CARTESIAN_POINT('',(31.295061332806,41.6915321010441,20.));
#9125=CARTESIAN_POINT('Origin',(28.795061332806,41.6915321010441,-20.));
#9126=CARTESIAN_POINT('Origin',(28.795061332806,-41.6915321010441,20.));
#9127=CARTESIAN_POINT('',(31.295061332806,-41.6915321010441,20.));
#9128=CARTESIAN_POINT('Origin',(28.795061332806,-41.6915321010441,20.));
#9129=CARTESIAN_POINT('',(31.295061332806,-41.6915321010441,1.76587979759228));
#9130=CARTESIAN_POINT('',(31.295061332806,-41.6915321010441,20.));
#9131=CARTESIAN_POINT('',(28.795061332806,-44.1915321010441,0.356833582029306));
#9132=CARTESIAN_POINT('Ctrl Pts',(28.795061332806,-44.1915321010441,0.356833582029284));
#9133=CARTESIAN_POINT('Ctrl Pts',(29.1123372354701,-44.1915321010441,0.356833582029283));
#9134=CARTESIAN_POINT('Ctrl Pts',(29.4431932108887,-44.1275251245074,0.406497032324425));
#9135=CARTESIAN_POINT('Ctrl Pts',(30.0405259238277,-43.8830970093849,0.584048414544644));
#9136=CARTESIAN_POINT('Ctrl Pts',(30.3077002103262,-43.7030327750914,0.710075190333896));
#9137=CARTESIAN_POINT('Ctrl Pts',(30.7537122028376,-43.2788343380328,0.982143846508312));
#9138=CARTESIAN_POINT('Ctrl Pts',(30.95523862548,-42.9955925725868,1.15080480840548));
#9139=CARTESIAN_POINT('Ctrl Pts',(31.2260895128688,-42.3675807949546,1.47762784261656));
#9140=CARTESIAN_POINT('Ctrl Pts',(31.295061332806,-42.0223600026362,1.63521545889971));
#9141=CARTESIAN_POINT('Ctrl Pts',(31.295061332806,-41.6915321010441,1.76587979759228));
#9142=CARTESIAN_POINT('Ctrl Pts',(31.295061332806,-41.6915321010441,1.76587979759228));
#9143=CARTESIAN_POINT('Ctrl Pts',(31.295061332806,-41.3866319916517,1.88630365231953));
#9144=CARTESIAN_POINT('Ctrl Pts',(31.2356009535887,-41.0538505476253,1.99948444500592));
#9145=CARTESIAN_POINT('Ctrl Pts',(30.9806651650377,-40.432164168516,2.17871269254273));
#9146=CARTESIAN_POINT('Ctrl Pts',(30.7848653879944,-40.14362590236,2.24556937536941));
#9147=CARTESIAN_POINT('Ctrl Pts',(30.3341320698251,-39.697227181252,2.33582555282254));
#9148=CARTESIAN_POINT('Ctrl Pts',(30.0547757695599,-39.5067960121042,2.36674372859812));
#9149=CARTESIAN_POINT('Ctrl Pts',(29.4416881336803,-39.2539459288562,2.40438278535118));
#9150=CARTESIAN_POINT('Ctrl Pts',(29.1080053010609,-39.1915321010441,2.41192340176922));
#9151=CARTESIAN_POINT('Ctrl Pts',(28.4821173645511,-39.1915321010441,2.41192340176922));
#9152=CARTESIAN_POINT('Ctrl Pts',(28.1484345319317,-39.2539459288562,2.40438278535118));
#9153=CARTESIAN_POINT('Ctrl Pts',(27.5353468960521,-39.5067960121042,2.36674372859812));
#9154=CARTESIAN_POINT('Ctrl Pts',(27.2559905957869,-39.697227181252,2.33582555282254));
#9155=CARTESIAN_POINT('Ctrl Pts',(26.8052572776176,-40.14362590236,2.24556937536941));
#9156=CARTESIAN_POINT('Ctrl Pts',(26.6094575005743,-40.432164168516,2.17871269254273));
#9157=CARTESIAN_POINT('Ctrl Pts',(26.3545217120232,-41.0538505476253,1.99948444500592));
#9158=CARTESIAN_POINT('Ctrl Pts',(26.295061332806,-41.3866319916517,1.88630365231953));
#9159=CARTESIAN_POINT('Ctrl Pts',(26.295061332806,-42.0223600026362,1.63521545889971));
#9160=CARTESIAN_POINT('Ctrl Pts',(26.3640331527432,-42.3675807949547,1.47762784261656));
#9161=CARTESIAN_POINT('Ctrl Pts',(26.634884040132,-42.9955925725868,1.15080480840548));
#9162=CARTESIAN_POINT('Ctrl Pts',(26.8364104627744,-43.2788343380328,0.982143846508312));
#9163=CARTESIAN_POINT('Ctrl Pts',(27.2824224552858,-43.7030327750914,0.710075190333895));
#9164=CARTESIAN_POINT('Ctrl Pts',(27.5495967417843,-43.8830970093849,0.584048414544644));
#9165=CARTESIAN_POINT('Ctrl Pts',(28.1469294547233,-44.1275251245074,0.406497032324426));
#9166=CARTESIAN_POINT('Ctrl Pts',(28.4777854301419,-44.1915321010441,0.356833582029285));
#9167=CARTESIAN_POINT('Ctrl Pts',(28.795061332806,-44.1915321010441,0.356833582029285));
#9168=CARTESIAN_POINT('Origin',(28.795061332806,-41.6915321010441,20.));
#9169=CARTESIAN_POINT('',(28.795061332806,-44.1915321010441,-16.3568335820293));
#9170=CARTESIAN_POINT('',(31.295061332806,-41.6915321010441,-17.7658797975923));
#9171=CARTESIAN_POINT('Ctrl Pts',(28.795061332806,-44.1915321010441,-16.3568335820293));
#9172=CARTESIAN_POINT('Ctrl Pts',(28.4777854301419,-44.1915321010441,-16.3568335820293));
#9173=CARTESIAN_POINT('Ctrl Pts',(28.1469294547233,-44.1275251245074,-16.4064970323244));
#9174=CARTESIAN_POINT('Ctrl Pts',(27.5495967417843,-43.8830970093849,-16.5840484145446));
#9175=CARTESIAN_POINT('Ctrl Pts',(27.2824224552858,-43.7030327750914,-16.7100751903339));
#9176=CARTESIAN_POINT('Ctrl Pts',(26.8364104627744,-43.2788343380328,-16.9821438465083));
#9177=CARTESIAN_POINT('Ctrl Pts',(26.634884040132,-42.9955925725868,-17.1508048084055));
#9178=CARTESIAN_POINT('Ctrl Pts',(26.3640331527432,-42.3675807949546,-17.4776278426165));
#9179=CARTESIAN_POINT('Ctrl Pts',(26.295061332806,-42.0223600026362,-17.6352154588997));
#9180=CARTESIAN_POINT('Ctrl Pts',(26.295061332806,-41.3866319916517,-17.8863036523195));
#9181=CARTESIAN_POINT('Ctrl Pts',(26.3545217120232,-41.0538505476253,-17.9994844450059));
#9182=CARTESIAN_POINT('Ctrl Pts',(26.6094575005743,-40.432164168516,-18.1787126925427));
#9183=CARTESIAN_POINT('Ctrl Pts',(26.8052572776176,-40.14362590236,-18.2455693753694));
#9184=CARTESIAN_POINT('Ctrl Pts',(27.2559905957869,-39.697227181252,-18.3358255528225));
#9185=CARTESIAN_POINT('Ctrl Pts',(27.5353468960521,-39.5067960121042,-18.3667437285981));
#9186=CARTESIAN_POINT('Ctrl Pts',(28.1484345319317,-39.2539459288562,-18.4043827853512));
#9187=CARTESIAN_POINT('Ctrl Pts',(28.4821173645511,-39.1915321010441,-18.4119234017692));
#9188=CARTESIAN_POINT('Ctrl Pts',(29.1080053010609,-39.1915321010441,-18.4119234017692));
#9189=CARTESIAN_POINT('Ctrl Pts',(29.4416881336803,-39.2539459288562,-18.4043827853512));
#9190=CARTESIAN_POINT('Ctrl Pts',(30.0547757695599,-39.5067960121042,-18.3667437285981));
#9191=CARTESIAN_POINT('Ctrl Pts',(30.3341320698251,-39.697227181252,-18.3358255528225));
#9192=CARTESIAN_POINT('Ctrl Pts',(30.7848653879944,-40.14362590236,-18.2455693753694));
#9193=CARTESIAN_POINT('Ctrl Pts',(30.9806651650377,-40.432164168516,-18.1787126925427));
#9194=CARTESIAN_POINT('Ctrl Pts',(31.2356009535887,-41.0538505476253,-17.9994844450059));
#9195=CARTESIAN_POINT('Ctrl Pts',(31.295061332806,-41.3866319916517,-17.8863036523195));
#9196=CARTESIAN_POINT('Ctrl Pts',(31.295061332806,-41.6915321010441,-17.7658797975923));
#9197=CARTESIAN_POINT('Ctrl Pts',(31.295061332806,-41.6915321010441,-17.7658797975923));
#9198=CARTESIAN_POINT('Ctrl Pts',(31.295061332806,-42.0223600026362,-17.6352154588997));
#9199=CARTESIAN_POINT('Ctrl Pts',(31.2260895128688,-42.3675807949546,-17.4776278426165));
#9200=CARTESIAN_POINT('Ctrl Pts',(30.95523862548,-42.9955925725868,-17.1508048084055));
#9201=CARTESIAN_POINT('Ctrl Pts',(30.7537122028376,-43.2788343380328,-16.9821438465083));
#9202=CARTESIAN_POINT('Ctrl Pts',(30.3077002103262,-43.7030327750914,-16.7100751903339));
#9203=CARTESIAN_POINT('Ctrl Pts',(30.0405259238277,-43.8830970093849,-16.5840484145446));
#9204=CARTESIAN_POINT('Ctrl Pts',(29.4431932108887,-44.1275251245074,-16.4064970323244));
#9205=CARTESIAN_POINT('Ctrl Pts',(29.11233723547,-44.1915321010441,-16.3568335820293));
#9206=CARTESIAN_POINT('Ctrl Pts',(28.795061332806,-44.1915321010441,-16.3568335820293));
#9207=CARTESIAN_POINT('',(31.295061332806,-41.6915321010441,-20.));
#9208=CARTESIAN_POINT('',(31.295061332806,-41.6915321010441,20.));
#9209=CARTESIAN_POINT('Origin',(28.795061332806,-41.6915321010441,-20.));
#9210=CARTESIAN_POINT('Origin',(-28.795061332806,41.6915321010441,20.));
#9211=CARTESIAN_POINT('',(-26.295061332806,41.6915321010441,20.));
#9212=CARTESIAN_POINT('Origin',(-28.795061332806,41.6915321010441,20.));
#9213=CARTESIAN_POINT('',(-26.295061332806,41.6915321010441,1.76587979759228));
#9214=CARTESIAN_POINT('',(-26.295061332806,41.6915321010441,20.));
#9215=CARTESIAN_POINT('',(-28.795061332806,44.1915321010441,0.356833582029306));
#9216=CARTESIAN_POINT('Ctrl Pts',(-28.795061332806,44.1915321010441,0.356833582029283));
#9217=CARTESIAN_POINT('Ctrl Pts',(-29.1123372354701,44.1915321010441,0.356833582029283));
#9218=CARTESIAN_POINT('Ctrl Pts',(-29.4431932108887,44.1275251245074,0.406497032324425));
#9219=CARTESIAN_POINT('Ctrl Pts',(-30.0405259238277,43.8830970093849,0.584048414544644));
#9220=CARTESIAN_POINT('Ctrl Pts',(-30.3077002103262,43.7030327750914,0.710075190333896));
#9221=CARTESIAN_POINT('Ctrl Pts',(-30.7537122028376,43.2788343380328,0.982143846508312));
#9222=CARTESIAN_POINT('Ctrl Pts',(-30.95523862548,42.9955925725868,1.15080480840548));
#9223=CARTESIAN_POINT('Ctrl Pts',(-31.2260895128688,42.3675807949546,1.47762784261656));
#9224=CARTESIAN_POINT('Ctrl Pts',(-31.295061332806,42.0223600026362,1.63521545889971));
#9225=CARTESIAN_POINT('Ctrl Pts',(-31.295061332806,41.3866319916517,1.88630365231953));
#9226=CARTESIAN_POINT('Ctrl Pts',(-31.2356009535887,41.0538505476253,1.99948444500592));
#9227=CARTESIAN_POINT('Ctrl Pts',(-30.9806651650377,40.432164168516,2.17871269254273));
#9228=CARTESIAN_POINT('Ctrl Pts',(-30.7848653879944,40.14362590236,2.24556937536941));
#9229=CARTESIAN_POINT('Ctrl Pts',(-30.3341320698251,39.697227181252,2.33582555282254));
#9230=CARTESIAN_POINT('Ctrl Pts',(-30.0547757695599,39.5067960121042,2.36674372859812));
#9231=CARTESIAN_POINT('Ctrl Pts',(-29.4416881336803,39.2539459288562,2.40438278535118));
#9232=CARTESIAN_POINT('Ctrl Pts',(-29.1080053010609,39.1915321010441,2.41192340176922));
#9233=CARTESIAN_POINT('Ctrl Pts',(-28.4821173645511,39.1915321010441,2.41192340176922));
#9234=CARTESIAN_POINT('Ctrl Pts',(-28.1484345319317,39.2539459288562,2.40438278535118));
#9235=CARTESIAN_POINT('Ctrl Pts',(-27.5353468960521,39.5067960121042,2.36674372859812));
#9236=CARTESIAN_POINT('Ctrl Pts',(-27.2559905957869,39.697227181252,2.33582555282254));
#9237=CARTESIAN_POINT('Ctrl Pts',(-26.8052572776176,40.14362590236,2.24556937536941));
#9238=CARTESIAN_POINT('Ctrl Pts',(-26.6094575005743,40.432164168516,2.17871269254273));
#9239=CARTESIAN_POINT('Ctrl Pts',(-26.3545217120232,41.0538505476253,1.99948444500592));
#9240=CARTESIAN_POINT('Ctrl Pts',(-26.295061332806,41.3866319916517,1.88630365231953));
#9241=CARTESIAN_POINT('Ctrl Pts',(-26.295061332806,41.6915321010441,1.76587979759227));
#9242=CARTESIAN_POINT('Ctrl Pts',(-26.295061332806,41.6915321010441,1.76587979759227));
#9243=CARTESIAN_POINT('Ctrl Pts',(-26.295061332806,42.0223600026362,1.63521545889971));
#9244=CARTESIAN_POINT('Ctrl Pts',(-26.3640331527432,42.3675807949547,1.47762784261656));
#9245=CARTESIAN_POINT('Ctrl Pts',(-26.634884040132,42.9955925725868,1.15080480840548));
#9246=CARTESIAN_POINT('Ctrl Pts',(-26.8364104627744,43.2788343380328,0.982143846508312));
#9247=CARTESIAN_POINT('Ctrl Pts',(-27.2824224552858,43.7030327750914,0.710075190333895));
#9248=CARTESIAN_POINT('Ctrl Pts',(-27.5495967417843,43.8830970093849,0.584048414544644));
#9249=CARTESIAN_POINT('Ctrl Pts',(-28.1469294547233,44.1275251245074,0.406497032324426));
#9250=CARTESIAN_POINT('Ctrl Pts',(-28.4777854301419,44.1915321010441,0.356833582029285));
#9251=CARTESIAN_POINT('Ctrl Pts',(-28.795061332806,44.1915321010441,0.356833582029285));
#9252=CARTESIAN_POINT('Origin',(-28.795061332806,41.6915321010441,20.));
#9253=CARTESIAN_POINT('',(-28.795061332806,44.1915321010441,-16.3568335820293));
#9254=CARTESIAN_POINT('',(-26.295061332806,41.6915321010441,-17.7658797975923));
#9255=CARTESIAN_POINT('Ctrl Pts',(-28.795061332806,44.1915321010441,-16.3568335820293));
#9256=CARTESIAN_POINT('Ctrl Pts',(-28.4777854301419,44.1915321010441,-16.3568335820293));
#9257=CARTESIAN_POINT('Ctrl Pts',(-28.1469294547233,44.1275251245074,-16.4064970323244));
#9258=CARTESIAN_POINT('Ctrl Pts',(-27.5495967417843,43.8830970093849,-16.5840484145446));
#9259=CARTESIAN_POINT('Ctrl Pts',(-27.2824224552858,43.7030327750914,-16.7100751903339));
#9260=CARTESIAN_POINT('Ctrl Pts',(-26.8364104627744,43.2788343380328,-16.9821438465083));
#9261=CARTESIAN_POINT('Ctrl Pts',(-26.634884040132,42.9955925725868,-17.1508048084055));
#9262=CARTESIAN_POINT('Ctrl Pts',(-26.3640331527432,42.3675807949546,-17.4776278426165));
#9263=CARTESIAN_POINT('Ctrl Pts',(-26.295061332806,42.0223600026362,-17.6352154588997));
#9264=CARTESIAN_POINT('Ctrl Pts',(-26.295061332806,41.6915321010441,-17.7658797975923));
#9265=CARTESIAN_POINT('Ctrl Pts',(-26.295061332806,41.6915321010441,-17.7658797975923));
#9266=CARTESIAN_POINT('Ctrl Pts',(-26.295061332806,41.3866319916517,-17.8863036523195));
#9267=CARTESIAN_POINT('Ctrl Pts',(-26.3545217120232,41.0538505476253,-17.9994844450059));
#9268=CARTESIAN_POINT('Ctrl Pts',(-26.6094575005743,40.432164168516,-18.1787126925427));
#9269=CARTESIAN_POINT('Ctrl Pts',(-26.8052572776176,40.14362590236,-18.2455693753694));
#9270=CARTESIAN_POINT('Ctrl Pts',(-27.2559905957869,39.697227181252,-18.3358255528225));
#9271=CARTESIAN_POINT('Ctrl Pts',(-27.5353468960521,39.5067960121042,-18.3667437285981));
#9272=CARTESIAN_POINT('Ctrl Pts',(-28.1484345319317,39.2539459288562,-18.4043827853512));
#9273=CARTESIAN_POINT('Ctrl Pts',(-28.4821173645511,39.1915321010441,-18.4119234017692));
#9274=CARTESIAN_POINT('Ctrl Pts',(-29.1080053010609,39.1915321010441,-18.4119234017692));
#9275=CARTESIAN_POINT('Ctrl Pts',(-29.4416881336803,39.2539459288562,-18.4043827853512));
#9276=CARTESIAN_POINT('Ctrl Pts',(-30.0547757695599,39.5067960121042,-18.3667437285981));
#9277=CARTESIAN_POINT('Ctrl Pts',(-30.3341320698251,39.697227181252,-18.3358255528225));
#9278=CARTESIAN_POINT('Ctrl Pts',(-30.7848653879944,40.14362590236,-18.2455693753694));
#9279=CARTESIAN_POINT('Ctrl Pts',(-30.9806651650377,40.432164168516,-18.1787126925427));
#9280=CARTESIAN_POINT('Ctrl Pts',(-31.2356009535887,41.0538505476253,-17.9994844450059));
#9281=CARTESIAN_POINT('Ctrl Pts',(-31.295061332806,41.3866319916517,-17.8863036523195));
#9282=CARTESIAN_POINT('Ctrl Pts',(-31.295061332806,42.0223600026362,-17.6352154588997));
#9283=CARTESIAN_POINT('Ctrl Pts',(-31.2260895128688,42.3675807949546,-17.4776278426165));
#9284=CARTESIAN_POINT('Ctrl Pts',(-30.95523862548,42.9955925725868,-17.1508048084055));
#9285=CARTESIAN_POINT('Ctrl Pts',(-30.7537122028376,43.2788343380328,-16.9821438465083));
#9286=CARTESIAN_POINT('Ctrl Pts',(-30.3077002103262,43.7030327750914,-16.7100751903339));
#9287=CARTESIAN_POINT('Ctrl Pts',(-30.0405259238277,43.8830970093849,-16.5840484145446));
#9288=CARTESIAN_POINT('Ctrl Pts',(-29.4431932108887,44.1275251245074,-16.4064970323244));
#9289=CARTESIAN_POINT('Ctrl Pts',(-29.11233723547,44.1915321010441,-16.3568335820293));
#9290=CARTESIAN_POINT('Ctrl Pts',(-28.795061332806,44.1915321010441,-16.3568335820293));
#9291=CARTESIAN_POINT('',(-26.295061332806,41.6915321010441,-20.));
#9292=CARTESIAN_POINT('',(-26.295061332806,41.6915321010441,20.));
#9293=CARTESIAN_POINT('Origin',(-28.795061332806,41.6915321010441,-20.));
#9294=CARTESIAN_POINT('Origin',(-40.,-30.7011310483684,-19.));
#9295=CARTESIAN_POINT('',(-40.,-30.7011310483684,-19.));
#9296=CARTESIAN_POINT('',(-40.,-31.7011310483684,-20.));
#9297=CARTESIAN_POINT('',(-40.,-5.77584828627628,5.92528276209211));
#9298=CARTESIAN_POINT('',(40.,-30.7011310483684,-19.));
#9299=CARTESIAN_POINT('',(-40.,-30.7011310483684,-19.));
#9300=CARTESIAN_POINT('',(40.,-31.7011310483684,-20.));
#9301=CARTESIAN_POINT('',(40.,-30.7758482862763,-19.0747172379079));
#9302=CARTESIAN_POINT('',(-20.,-31.7011310483684,-20.));
#9303=CARTESIAN_POINT('Origin',(-40.,-11.9332887764186,-19.));
#9304=CARTESIAN_POINT('',(-40.,-11.9332887764186,-19.));
#9305=CARTESIAN_POINT('',(-40.,19.0333556117907,-19.));
#9306=CARTESIAN_POINT('',(40.,-11.9332887764186,-19.));
#9307=CARTESIAN_POINT('',(-40.,-11.9332887764186,-19.));
#9308=CARTESIAN_POINT('',(40.,-30.9666443882093,-19.));
#9309=CARTESIAN_POINT('Origin',(-40.,-10.9332887764186,-20.));
#9310=CARTESIAN_POINT('',(-40.,-10.9332887764186,-20.));
#9311=CARTESIAN_POINT('',(-40.,-0.699966582313925,-30.2333221941047));
#9312=CARTESIAN_POINT('',(40.,-10.9332887764186,-20.));
#9313=CARTESIAN_POINT('',(-20.,-10.9332887764186,-20.));
#9314=CARTESIAN_POINT('',(40.,-25.6999665823139,-5.23332219410464));
#9315=CARTESIAN_POINT('Origin',(-8.88178419700125E-15,8.88178419700125E-15,
-20.));
#9316=CARTESIAN_POINT('',(40.,-47.,-20.));
#9317=CARTESIAN_POINT('',(40.,50.,-20.));
#9318=CARTESIAN_POINT('',(-40.,-47.,-20.));
#9319=CARTESIAN_POINT('',(-20.,-47.,-20.));
#9320=CARTESIAN_POINT('',(-40.,-50.,-20.));
#9321=CARTESIAN_POINT('Origin',(-8.88178419700125E-15,8.88178419700125E-15,
-20.));
#9322=CARTESIAN_POINT('',(-40.,10.9332887764186,-20.));
#9323=CARTESIAN_POINT('',(-40.,-50.,-20.));
#9324=CARTESIAN_POINT('',(40.,10.9332887764186,-20.));
#9325=CARTESIAN_POINT('',(-20.,10.9332887764186,-20.));
#9326=CARTESIAN_POINT('',(40.,50.,-20.));
#9327=CARTESIAN_POINT('Origin',(-40.,50.,0.));
#9328=CARTESIAN_POINT('',(-40.,-50.,-17.));
#9329=CARTESIAN_POINT('',(-40.,-28.5,-38.5));
#9330=CARTESIAN_POINT('',(-40.,-50.,17.));
#9331=CARTESIAN_POINT('',(-40.,-50.,0.));
#9332=CARTESIAN_POINT('',(-40.,-47.,20.));
#9333=CARTESIAN_POINT('',(-40.,-28.5,38.5));
#9334=CARTESIAN_POINT('',(-40.,-31.7011310483684,20.));
#9335=CARTESIAN_POINT('',(-40.,-50.,20.));
#9336=CARTESIAN_POINT('',(-40.,-30.7011310483684,19.));
#9337=CARTESIAN_POINT('',(-40.,-5.77584828627628,-5.92528276209211));
#9338=CARTESIAN_POINT('',(-40.,-11.9332887764186,19.));
#9339=CARTESIAN_POINT('',(-40.,19.0333556117907,19.));
#9340=CARTESIAN_POINT('',(-40.,-10.9332887764186,20.));
#9341=CARTESIAN_POINT('',(-40.,-0.699966582313925,30.2333221941047));
#9342=CARTESIAN_POINT('',(-40.,10.9332887764186,20.));
#9343=CARTESIAN_POINT('',(-40.,-50.,20.));
#9344=CARTESIAN_POINT('',(-40.,11.9332887764186,19.));
#9345=CARTESIAN_POINT('',(-40.,25.6999665823139,5.23332219410463));
#9346=CARTESIAN_POINT('',(-40.,30.7011310483684,19.));
#9347=CARTESIAN_POINT('',(-40.,30.9666443882093,19.));
#9348=CARTESIAN_POINT('',(-40.,31.7011310483684,20.));
#9349=CARTESIAN_POINT('',(-40.,30.7758482862763,19.0747172379079));
#9350=CARTESIAN_POINT('',(-40.,47.,20.));
#9351=CARTESIAN_POINT('',(-40.,-50.,20.));
#9352=CARTESIAN_POINT('',(-40.,50.,17.));
#9353=CARTESIAN_POINT('',(-40.,53.5,13.5));
#9354=CARTESIAN_POINT('',(-40.,50.,-17.));
#9355=CARTESIAN_POINT('',(-40.,50.,0.));
#9356=CARTESIAN_POINT('',(-40.,47.,-20.));
#9357=CARTESIAN_POINT('',(-40.,53.5,-13.5));
#9358=CARTESIAN_POINT('',(-40.,31.7011310483684,-20.));
#9359=CARTESIAN_POINT('',(-40.,-50.,-20.));
#9360=CARTESIAN_POINT('',(-40.,30.7011310483684,-19.));
#9361=CARTESIAN_POINT('',(-40.,30.7758482862763,-19.0747172379079));
#9362=CARTESIAN_POINT('',(-40.,11.9332887764186,-19.));
#9363=CARTESIAN_POINT('',(-40.,30.9666443882093,-19.));
#9364=CARTESIAN_POINT('',(-40.,25.6999665823139,-5.23332219410463));
#9365=CARTESIAN_POINT('',(-40.,48.3343839603864,-7.99999999999999));
#9366=CARTESIAN_POINT('Origin',(-40.,37.8343839603864,-7.99999999999999));
#9367=CARTESIAN_POINT('',(-40.,-48.3343839603864,-7.99999999999999));
#9368=CARTESIAN_POINT('Origin',(-40.,-37.8343839603864,-7.99999999999999));
#9369=CARTESIAN_POINT('',(-40.,-17.5,8.38733349006174E-15));
#9370=CARTESIAN_POINT('Origin',(-40.,1.91963385766348E-15,1.05304653885696E-14));
#9371=CARTESIAN_POINT('Origin',(-40.,30.7011310483684,-19.));
#9372=CARTESIAN_POINT('',(40.,31.7011310483684,-20.));
#9373=CARTESIAN_POINT('',(-20.,31.7011310483684,-20.));
#9374=CARTESIAN_POINT('',(40.,30.7011310483684,-19.));
#9375=CARTESIAN_POINT('',(40.,5.77584828627629,5.9252827620921));
#9376=CARTESIAN_POINT('',(-40.,30.7011310483684,-19.));
#9377=CARTESIAN_POINT('Origin',(-40.,11.9332887764186,-19.));
#9378=CARTESIAN_POINT('',(40.,11.9332887764186,-19.));
#9379=CARTESIAN_POINT('',(40.,-19.0333556117907,-19.));
#9380=CARTESIAN_POINT('',(-40.,11.9332887764186,-19.));
#9381=CARTESIAN_POINT('Origin',(-40.,10.9332887764186,-20.));
#9382=CARTESIAN_POINT('',(40.,0.699966582313925,-30.2333221941046));
#9383=CARTESIAN_POINT('Origin',(40.,-50.,0.));
#9384=CARTESIAN_POINT('',(40.,47.,-20.));
#9385=CARTESIAN_POINT('',(40.,50.,-20.));
#9386=CARTESIAN_POINT('',(40.,50.,-17.));
#9387=CARTESIAN_POINT('',(40.,28.5,-38.5));
#9388=CARTESIAN_POINT('',(40.,50.,17.));
#9389=CARTESIAN_POINT('',(40.,50.,0.));
#9390=CARTESIAN_POINT('',(40.,47.,20.));
#9391=CARTESIAN_POINT('',(40.,28.5,38.5));
#9392=CARTESIAN_POINT('',(40.,31.7011310483684,20.));
#9393=CARTESIAN_POINT('',(40.,50.,20.));
#9394=CARTESIAN_POINT('',(40.,30.7011310483684,19.));
#9395=CARTESIAN_POINT('',(40.,5.77584828627629,-5.9252827620921));
#9396=CARTESIAN_POINT('',(40.,11.9332887764186,19.));
#9397=CARTESIAN_POINT('',(40.,-19.0333556117907,19.));
#9398=CARTESIAN_POINT('',(40.,10.9332887764186,20.));
#9399=CARTESIAN_POINT('',(40.,0.699966582313925,30.2333221941046));
#9400=CARTESIAN_POINT('',(40.,-10.9332887764186,20.));
#9401=CARTESIAN_POINT('',(40.,50.,20.));
#9402=CARTESIAN_POINT('',(40.,-11.9332887764186,19.));
#9403=CARTESIAN_POINT('',(40.,-25.6999665823139,5.23332219410464));
#9404=CARTESIAN_POINT('',(40.,-30.7011310483684,19.));
#9405=CARTESIAN_POINT('',(40.,-30.9666443882093,19.));
#9406=CARTESIAN_POINT('',(40.,-31.7011310483684,20.));
#9407=CARTESIAN_POINT('',(40.,-30.7758482862763,19.0747172379079));
#9408=CARTESIAN_POINT('',(40.,-47.,20.));
#9409=CARTESIAN_POINT('',(40.,50.,20.));
#9410=CARTESIAN_POINT('',(40.,-50.,17.));
#9411=CARTESIAN_POINT('',(40.,-53.5,13.5));
#9412=CARTESIAN_POINT('',(40.,-50.,-17.));
#9413=CARTESIAN_POINT('',(40.,-50.,0.));
#9414=CARTESIAN_POINT('',(40.,-53.5,-13.5));
#9415=CARTESIAN_POINT('',(40.,48.3343839603864,-7.99999999999999));
#9416=CARTESIAN_POINT('Origin',(40.,37.8343839603864,-7.99999999999999));
#9417=CARTESIAN_POINT('',(40.,-48.3343839603864,-7.99999999999999));
#9418=CARTESIAN_POINT('Origin',(40.,-37.8343839603864,-7.99999999999999));
#9419=CARTESIAN_POINT('',(40.,-17.5,8.38733349006174E-15));
#9420=CARTESIAN_POINT('Origin',(40.,1.91963385766348E-15,1.05304653885696E-14));
#9421=CARTESIAN_POINT('Origin',(-8.88178419700125E-15,8.88178419700125E-15,
-20.));
#9422=CARTESIAN_POINT('',(20.,47.,-20.));
#9423=CARTESIAN_POINT('Origin',(-40.,-30.7011310483684,19.));
#9424=CARTESIAN_POINT('',(-20.,-31.7011310483684,20.));
#9425=CARTESIAN_POINT('',(-40.,-30.7011310483684,19.));
#9426=CARTESIAN_POINT('Origin',(-40.,-11.9332887764186,19.));
#9427=CARTESIAN_POINT('',(-40.,-11.9332887764186,19.));
#9428=CARTESIAN_POINT('Origin',(-40.,-10.9332887764186,20.));
#9429=CARTESIAN_POINT('',(-20.,-10.9332887764186,20.));
#9430=CARTESIAN_POINT('Origin',(-8.88178419700125E-15,8.88178419700125E-15,
20.));
#9431=CARTESIAN_POINT('',(-20.,-47.,20.));
#9432=CARTESIAN_POINT('Origin',(-8.88178419700125E-15,8.88178419700125E-15,
20.));
#9433=CARTESIAN_POINT('',(-20.,10.9332887764186,20.));
#9434=CARTESIAN_POINT('Origin',(-40.,30.7011310483684,19.));
#9435=CARTESIAN_POINT('',(-40.,30.7011310483684,19.));
#9436=CARTESIAN_POINT('',(-20.,31.7011310483684,20.));
#9437=CARTESIAN_POINT('Origin',(-40.,11.9332887764186,19.));
#9438=CARTESIAN_POINT('',(-40.,11.9332887764186,19.));
#9439=CARTESIAN_POINT('Origin',(-40.,10.9332887764186,20.));
#9440=CARTESIAN_POINT('Origin',(-8.88178419700125E-15,8.88178419700125E-15,
20.));
#9441=CARTESIAN_POINT('',(20.,47.,20.));
#9442=CARTESIAN_POINT('Origin',(0.,37.8343839603864,-7.99999999999999));
#9443=CARTESIAN_POINT('',(0.,48.3343839603864,-7.99999999999999));
#9444=CARTESIAN_POINT('Origin',(0.,-37.8343839603864,-7.99999999999999));
#9445=CARTESIAN_POINT('',(0.,-48.3343839603864,-7.99999999999999));
#9446=CARTESIAN_POINT('Origin',(0.,1.91963385766348E-15,1.05304653885696E-14));
#9447=CARTESIAN_POINT('',(0.,-17.5,1.26735972870775E-14));
#9448=CARTESIAN_POINT('Origin',(20.,48.5,-18.5));
#9449=CARTESIAN_POINT('',(20.,50.,-17.));
#9450=CARTESIAN_POINT('Origin',(40.,50.,0.));
#9451=CARTESIAN_POINT('',(20.,50.,17.));
#9452=CARTESIAN_POINT('Origin',(20.,48.5,18.5));
#9453=CARTESIAN_POINT('Origin',(-20.,-48.5,-18.5));
#9454=CARTESIAN_POINT('',(-20.,-50.,-17.));
#9455=CARTESIAN_POINT('Origin',(-40.,-50.,0.));
#9456=CARTESIAN_POINT('',(-20.,-50.,17.));
#9457=CARTESIAN_POINT('Origin',(-20.,-48.5,18.5));
#9484=UNCERTAINTY_MEASURE_WITH_UNIT(LENGTH_MEASURE(0.01),#9497,
'DISTANCE_ACCURACY_VALUE',
'Maximum model space distance between geometric entities at asserted c
onnectivities');
#9485=UNCERTAINTY_MEASURE_WITH_UNIT(LENGTH_MEASURE(0.01),#9497,
'DISTANCE_ACCURACY_VALUE',
'Maximum model space distance between geometric entities at asserted c
onnectivities');
#9495=(
GEOMETRIC_REPRESENTATION_CONTEXT(3)
GLOBAL_UNCERTAINTY_ASSIGNED_CONTEXT((#9484))
GLOBAL_UNIT_ASSIGNED_CONTEXT((#9497,#9499,#9500))
REPRESENTATION_CONTEXT('','3D')
);
#9496=(
GEOMETRIC_REPRESENTATION_CONTEXT(3)
GLOBAL_UNCERTAINTY_ASSIGNED_CONTEXT((#9485))
GLOBAL_UNIT_ASSIGNED_CONTEXT((#9497,#9499,#9500))
REPRESENTATION_CONTEXT('','3D')
);
#9497=(
LENGTH_UNIT()
NAMED_UNIT(*)
SI_UNIT(.MILLI.,.METRE.)
);
#9499=(
NAMED_UNIT(*)
PLANE_ANGLE_UNIT()
SI_UNIT($,.RADIAN.)
);
#9500=(
NAMED_UNIT(*)
SI_UNIT($,.STERADIAN.)
SOLID_ANGLE_UNIT()
);
#9510=SHAPE_DEFINITION_REPRESENTATION(#9520,#9547);
#9520=PRODUCT_DEFINITION_SHAPE('',$,#9558);
#9547=SHAPE_REPRESENTATION('',(#5757),#9495);
#9548=PRODUCT_DEFINITION_CONTEXT('part definition',#9580,'design');
#9558=PRODUCT_DEFINITION('Slide_Block','Slide_Block',#9568,#9548);
#9568=PRODUCT_DEFINITION_FORMATION('',$,#9591);
#9580=APPLICATION_CONTEXT(
'Core Data for Automotive Mechanical Design Process');
#9581=PRODUCT_CONTEXT('part definition',#9580,'mechanical');
#9591=PRODUCT('Slide_Block','Slide_Block',$,(#9581));
#9593=PRESENTATION_STYLE_ASSIGNMENT((#9596));
#9596=SURFACE_STYLE_USAGE(.BOTH.,#9599);
#9599=SURFACE_SIDE_STYLE('',(#9602));
#9602=SURFACE_STYLE_FILL_AREA(#9605);
#9605=FILL_AREA_STYLE('Opaque(245,245,246)',(#9608));
#9608=FILL_AREA_STYLE_COLOUR('Opaque(245,245,246)',#9611);
#9611=COLOUR_RGB('Opaque(245,245,246)', 0.66274510, 0.83137255, 0.94901961);
ENDSEC;
END-ISO-10303-21;
